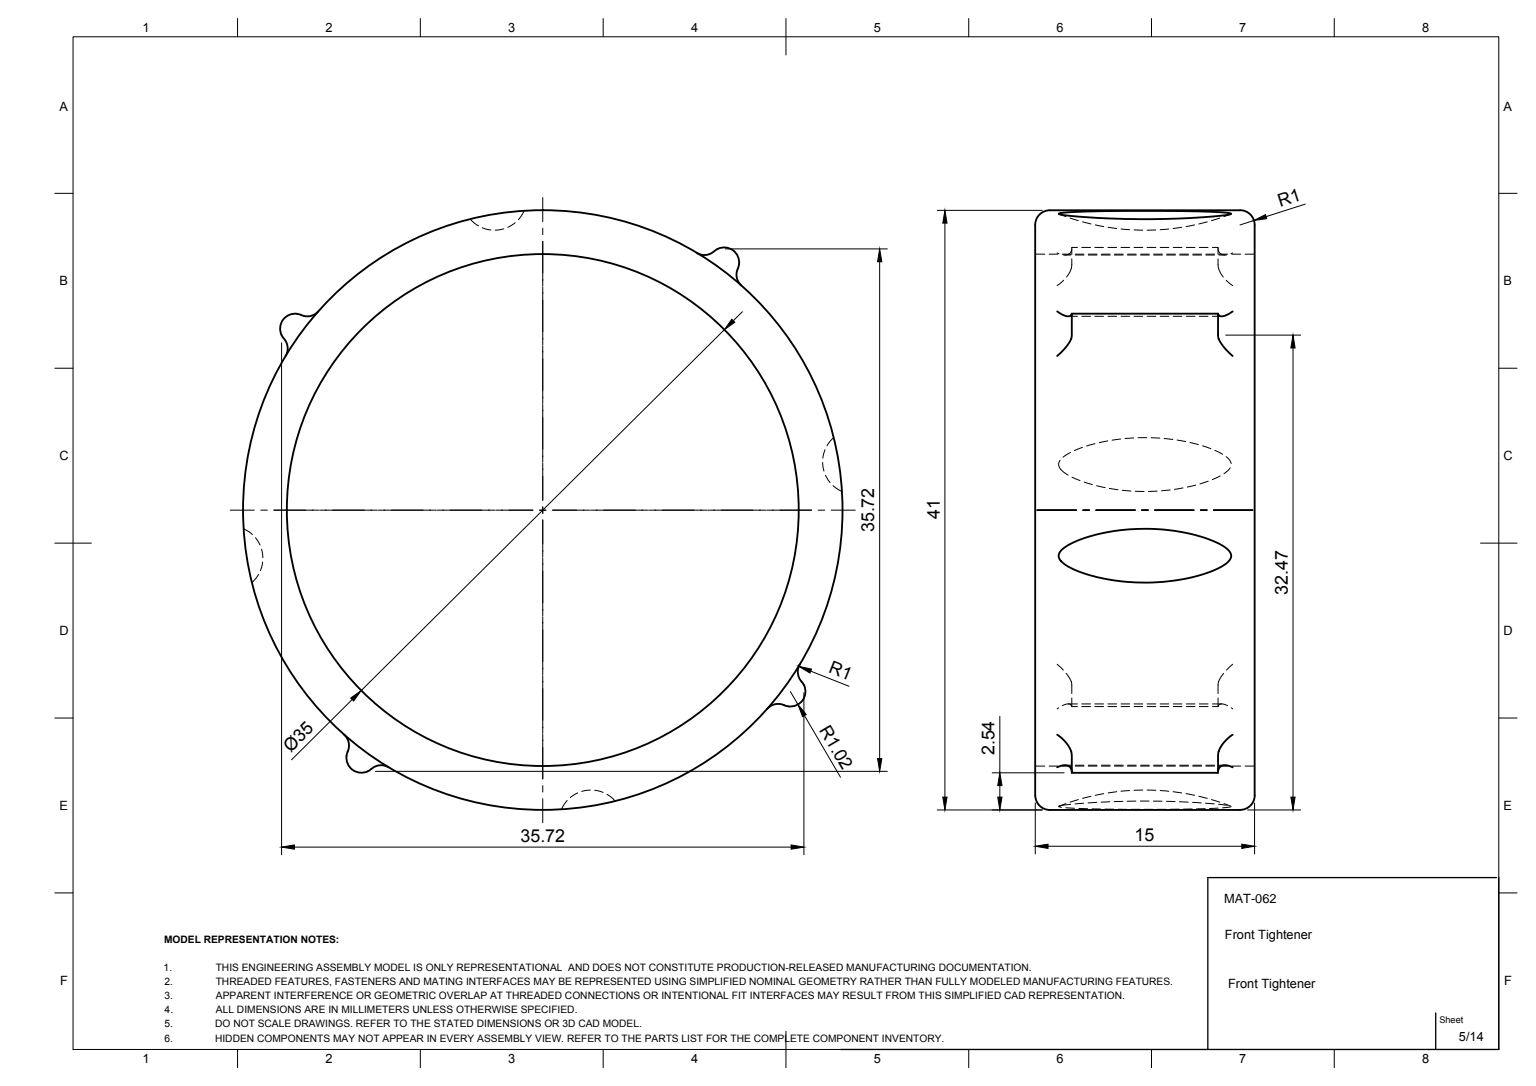
ISO-10303-21;
HEADER;
/* Generated by software containing ST-Developer
 * from STEP Tools, Inc. (www.steptools.com) 
 */

FILE_DESCRIPTION(
/* description */ (''),
/* implementation_level */ '2;1');

FILE_NAME(
/* name */ 'Front Tightener.step',
/* time_stamp */ '2026-10-24T10:18:25-07:00',
/* author */ (''),
/* organization */ (''),
/* preprocessor_version */ 'ST-DEVELOPER v20.2',
/* originating_system */ 'Autodesk Translation Framework v15.15.0.0',
/* authorisation */ '');

FILE_SCHEMA (('AUTOMOTIVE_DESIGN { 1 0 10303 214 3 1 1 }'));
ENDSEC;

DATA;
#10=MECHANICAL_DESIGN_GEOMETRIC_PRESENTATION_REPRESENTATION('',(#249),#14125);
#209=TOROIDAL_SURFACE('',#6436,21.5,1.);
#210=TOROIDAL_SURFACE('',#6437,21.5,1.);
#211=TOROIDAL_SURFACE('',#6461,21.5,1.);
#212=TOROIDAL_SURFACE('',#6462,21.5,1.);
#213=TOROIDAL_SURFACE('',#6465,21.5,1.);
#214=TOROIDAL_SURFACE('',#6466,21.5,1.);
#215=TOROIDAL_SURFACE('',#6469,21.5,1.);
#216=TOROIDAL_SURFACE('',#6470,21.5,1.);
#217=TOROIDAL_SURFACE('',#6472,19.5,1.);
#218=TOROIDAL_SURFACE('',#6474,19.5,1.);
#223=(
BOUNDED_SURFACE()
B_SPLINE_SURFACE(2,2,((#11091,#11092,#11093,#11094,#11095),(#11096,#11097,
#11098,#11099,#11100),(#11101,#11102,#11103,#11104,#11105)),
 .UNSPECIFIED.,.F.,.F.,.F.)
B_SPLINE_SURFACE_WITH_KNOTS((3,3),(3,2,3),(-0.372145961557786,0.372122372471418),
(-2.5862005619648,-1.57539112175776,-0.564581681550713),.UNSPECIFIED.)
GEOMETRIC_REPRESENTATION_ITEM()
RATIONAL_B_SPLINE_SURFACE(((1.,0.874978596158143,1.,0.874978596158143,1.),
(0.931553475244656,0.815089352015808,0.931553475244656,0.815089352015808,
0.931553475244656),(1.,0.874978596158143,1.,0.874978596158143,1.)))
REPRESENTATION_ITEM('')
SURFACE()
);
#224=(
BOUNDED_SURFACE()
B_SPLINE_SURFACE(2,2,((#11106,#11107,#11108,#11109,#11110),(#11111,#11112,
#11113,#11114,#11115),(#11116,#11117,#11118,#11119,#11120)),
 .UNSPECIFIED.,.F.,.F.,.F.)
B_SPLINE_SURFACE_WITH_KNOTS((3,3),(3,2,3),(-0.372145961557785,0.372122372471416),
(-1.01540423516984,-0.00459479496282911,1.00621464524418),.UNSPECIFIED.)
GEOMETRIC_REPRESENTATION_ITEM()
RATIONAL_B_SPLINE_SURFACE(((1.,0.874978596158151,1.,0.874978596158151,1.),
(0.931553475244656,0.815089352015816,0.931553475244656,0.815089352015816,
0.931553475244656),(1.,0.874978596158151,1.,0.874978596158151,1.)))
REPRESENTATION_ITEM('')
SURFACE()
);
#225=(
BOUNDED_SURFACE()
B_SPLINE_SURFACE(2,2,((#11121,#11122,#11123,#11124,#11125),(#11126,#11127,
#11128,#11129,#11130),(#11131,#11132,#11133,#11134,#11135)),
 .UNSPECIFIED.,.F.,.F.,.F.)
B_SPLINE_SURFACE_WITH_KNOTS((3,3),(3,2,3),(-0.372145961557786,0.372122372471418),
(0.555392091624955,1.56620153183202,2.57701097203908),.UNSPECIFIED.)
GEOMETRIC_REPRESENTATION_ITEM()
RATIONAL_B_SPLINE_SURFACE(((1.,0.874978596158138,1.,0.874978596158138,1.),
(0.931553475244654,0.815089352015803,0.931553475244654,0.815089352015803,
0.931553475244654),(1.,0.874978596158138,1.,0.874978596158138,1.)))
REPRESENTATION_ITEM('')
SURFACE()
);
#226=(
BOUNDED_SURFACE()
B_SPLINE_SURFACE(2,2,((#11136,#11137,#11138,#11139,#11140),(#11141,#11142,
#11143,#11144,#11145),(#11146,#11147,#11148,#11149,#11150)),
 .UNSPECIFIED.,.F.,.F.,.F.)
B_SPLINE_SURFACE_WITH_KNOTS((3,3),(3,2,3),(-0.371934671474245,0.371934671474244),
(-1.01080944020701,0.,1.01080944020701),.UNSPECIFIED.)
GEOMETRIC_REPRESENTATION_ITEM()
RATIONAL_B_SPLINE_SURFACE(((1.,0.87497859615815,1.,0.87497859615815,1.),
(0.93162599415309,0.815152804508512,0.93162599415309,0.815152804508512,
0.93162599415309),(1.,0.87497859615815,1.,0.87497859615815,1.)))
REPRESENTATION_ITEM('')
SURFACE()
);
#229=SHAPE_REPRESENTATION_RELATIONSHIP('SRR','None',#14202,#239);
#239=ADVANCED_BREP_SHAPE_REPRESENTATION('',(#268),#14116);
#249=STYLED_ITEM('',(#14263),#268);
#268=MANIFOLD_SOLID_BREP('Front Tightener',#6136);
#357=B_SPLINE_CURVE_WITH_KNOTS('',3,(#10853,#10854,#10855,#10856,#10857,
#10858,#10859,#10860),.UNSPECIFIED.,.F.,.F.,(4,2,2,4),(-1.01270550863141,
-0.972225883052009,-0.93592471729076,-0.9302261633243),.UNSPECIFIED.);
#358=B_SPLINE_CURVE_WITH_KNOTS('',3,(#10862,#10863,#10864,#10865,#10866,
#10867,#10868,#10869,#10870,#10871,#10872,#10873,#10874,#10875,#10876,#10877,
#10878,#10879,#10880,#10881,#10882,#10883),.UNSPECIFIED.,.F.,.F.,(4,2,2,
2,2,2,2,2,2,2,4),(0.770301299294677,0.776837516381544,0.810179859704117,
0.863854547164407,0.965601485426607,1.16658222290299,1.71041595764289,2.04547866914785,
2.21675572625692,2.31744906128486,2.32707423972487),.UNSPECIFIED.);
#359=B_SPLINE_CURVE_WITH_KNOTS('',3,(#10889,#10890,#10891,#10892,#10893,
#10894,#10895,#10896,#10897,#10898,#10899,#10900,#10901,#10902,#10903,#10904,
#10905,#10906,#10907,#10908,#10909,#10910,#10911,#10912,#10913),
 .UNSPECIFIED.,.F.,.F.,(4,2,2,2,2,3,2,2,2,2,2,4),(-0.9302261633243,-0.897559179923855,
-0.841033612998941,-0.72014052841894,-0.534875041413907,0.,0.287237711284631,
0.543909079429507,0.657892073847931,0.715678915934471,0.748705009105826,
0.770301299294677),.UNSPECIFIED.);
#360=B_SPLINE_CURVE_WITH_KNOTS('',3,(#10947,#10948,#10949,#10950,#10951,
#10952,#10953,#10954,#10955,#10956,#10957,#10958,#10959,#10960,#10961,#10962,
#10963,#10964,#10965,#10966,#10967,#10968,#10969,#10970,#10971,#10972,#10973,
#10974,#10975,#10976,#10977,#10978,#10979,#10980,#10981,#10982,#10983,#10984,
#10985,#10986,#10987,#10988,#10989,#10990),.UNSPECIFIED.,.T.,.F.,(4,2,2,
2,2,2,2,2,2,2,2,2,2,2,2,2,2,2,2,2,2,4),(-3.33977974833692,-3.05254203705232,
-2.79587066890727,-2.68188767448872,-2.62410083240212,-2.59107473923068,
-2.56294223195498,-2.52959988863245,-2.47592520117237,-2.37417826291126,
-2.17319752543706,-1.62936379070288,-1.29430107920164,-1.12302402209434,
-1.02233068706724,-0.972225883048282,-0.935924717287512,-0.897559179921191,
-0.841033612997187,-0.720140528418584,-0.534875041413949,0.),
 .UNSPECIFIED.);
#361=B_SPLINE_CURVE_WITH_KNOTS('',3,(#10992,#10993,#10994,#10995,#10996,
#10997,#10998,#10999,#11000,#11001,#11002,#11003,#11004,#11005,#11006,#11007,
#11008,#11009,#11010,#11011,#11012,#11013,#11014,#11015,#11016,#11017,#11018,
#11019,#11020,#11021,#11022,#11023,#11024,#11025,#11026,#11027,#11028,#11029,
#11030,#11031,#11032,#11033,#11034,#11035),.UNSPECIFIED.,.T.,.F.,(4,2,2,
2,2,2,2,2,2,2,2,2,2,2,2,2,2,2,2,2,2,4),(-3.3397797483622,-3.05254203707762,
-2.79587066893242,-2.68188767451365,-2.62410083242683,-2.5910747392553,
-2.5629422319795,-2.52959988865681,-2.47592520119621,-2.37417826293345,
-2.17319752545607,-1.62936379071395,-1.29430107920719,-1.1230240220981,
-1.02233068707054,-0.972225883051298,-0.93592471729009,-0.89755917992317,
-0.841033612998203,-0.720140528418294,-0.534875041413579,0.),
 .UNSPECIFIED.);
#362=B_SPLINE_CURVE_WITH_KNOTS('',3,(#11037,#11038,#11039,#11040,#11041,
#11042,#11043,#11044,#11045,#11046,#11047,#11048,#11049,#11050,#11051,#11052,
#11053,#11054,#11055,#11056,#11057,#11058,#11059,#11060,#11061,#11062,#11063,
#11064,#11065,#11066,#11067,#11068,#11069,#11070,#11071,#11072,#11073,#11074,
#11075,#11076,#11077,#11078,#11079,#11080),.UNSPECIFIED.,.T.,.F.,(4,2,2,
2,2,2,2,2,2,2,2,2,2,2,2,2,2,2,2,2,2,4),(-3.3397797483903,-3.05254203710569,
-2.79587066896086,-2.68188767454252,-2.62410083245608,-2.59107473928483,
-2.56294223200934,-2.52959988868709,-2.47592520122646,-2.37417826296174,
-2.17319752548078,-1.62936379072977,-1.29430107921846,-1.12302402210607,
-1.02233068707609,-0.972225883055856,-0.935924717293985,-0.897559179926439,
-0.841033613000712,-0.720140528419696,-0.534875041414283,0.),
 .UNSPECIFIED.);
#363=B_SPLINE_CURVE_WITH_KNOTS('',3,(#11156,#11157,#11158,#11159,#11160,
#11161),.UNSPECIFIED.,.F.,.F.,(4,2,4),(0.661047189651573,0.682893822496354,
0.69260663288377),.UNSPECIFIED.);
#364=B_SPLINE_CURVE_WITH_KNOTS('',3,(#11165,#11166,#11167,#11168,#11169,
#11170),.UNSPECIFIED.,.F.,.F.,(4,2,4),(0.954385955540414,0.955688960187291,
0.983990255335198),.UNSPECIFIED.);
#365=B_SPLINE_CURVE_WITH_KNOTS('',3,(#11174,#11175,#11176,#11177,#11178,
#11179),.UNSPECIFIED.,.F.,.F.,(4,2,4),(0.11431583352954,0.135832218753253,
0.145774815807224),.UNSPECIFIED.);
#366=B_SPLINE_CURVE_WITH_KNOTS('',3,(#11182,#11183,#11184,#11185,#11186,
#11187),.UNSPECIFIED.,.F.,.F.,(4,2,4),(0.406957049146252,0.408029153839697,
0.43652027355868),.UNSPECIFIED.);
#367=B_SPLINE_CURVE_WITH_KNOTS('',3,(#11193,#11194,#11195,#11196,#11197,
#11198,#11199,#11200,#11201,#11202),.UNSPECIFIED.,.F.,.F.,(4,2,2,2,4),(-0.178698063821344,
-0.13526955955559,-0.076624980274606,0.,0.000624348927189005),
 .UNSPECIFIED.);
#368=B_SPLINE_CURVE_WITH_KNOTS('',3,(#11203,#11204,#11205,#11206,#11207,
#11208,#11209,#11210,#11211,#11212),.UNSPECIFIED.,.F.,.F.,(4,2,2,2,4),(0.221433756193381,
0.257003031040665,0.305034737267452,0.367792942517405,0.3683043034075),
 .UNSPECIFIED.);
#369=B_SPLINE_CURVE_WITH_KNOTS('',3,(#11214,#11215,#11216,#11217,#11218,
#11219,#11220,#11221,#11222,#11223),.UNSPECIFIED.,.F.,.F.,(4,2,2,2,4),(-0.178698063657826,
-0.135269559443281,-0.0766249802302674,0.,0.000624348926984052),
 .UNSPECIFIED.);
#370=B_SPLINE_CURVE_WITH_KNOTS('',3,(#11225,#11226,#11227,#11228,#11229,
#11230,#11231,#11232,#11233,#11234),.UNSPECIFIED.,.F.,.F.,(4,2,2,2,4),(0.22143375619356,
0.257003031040236,0.305034737266783,0.367792942534155,0.36830430342492),
 .UNSPECIFIED.);
#371=B_SPLINE_CURVE_WITH_KNOTS('',3,(#11241,#11242,#11243,#11244,#11245,
#11246),.UNSPECIFIED.,.F.,.F.,(4,2,4),(0.661047189631137,0.682893822475484,
0.692606632862655),.UNSPECIFIED.);
#372=B_SPLINE_CURVE_WITH_KNOTS('',3,(#11250,#11251,#11252,#11253,#11254,
#11255),.UNSPECIFIED.,.F.,.F.,(4,2,4),(0.954385955875588,0.955688960523108,
0.983990255684603),.UNSPECIFIED.);
#373=B_SPLINE_CURVE_WITH_KNOTS('',3,(#11259,#11260,#11261,#11262,#11263,
#11264),.UNSPECIFIED.,.F.,.F.,(4,2,4),(0.11431583355748,0.135832218786672,
0.145774815843186),.UNSPECIFIED.);
#374=B_SPLINE_CURVE_WITH_KNOTS('',3,(#11267,#11268,#11269,#11270,#11271,
#11272),.UNSPECIFIED.,.F.,.F.,(4,2,4),(0.406957049130622,0.408029153824045,
0.436520273542523),.UNSPECIFIED.);
#375=B_SPLINE_CURVE_WITH_KNOTS('',3,(#11282,#11283,#11284,#11285,#11286,
#11287),.UNSPECIFIED.,.F.,.F.,(4,2,4),(0.661047189621191,0.682893822464398,
0.692606632851314),.UNSPECIFIED.);
#376=B_SPLINE_CURVE_WITH_KNOTS('',3,(#11291,#11292,#11293,#11294,#11295,
#11296),.UNSPECIFIED.,.F.,.F.,(4,2,4),(0.954385955650832,0.95568896029806,
0.983990255452134),.UNSPECIFIED.);
#377=B_SPLINE_CURVE_WITH_KNOTS('',3,(#11300,#11301,#11302,#11303,#11304,
#11305),.UNSPECIFIED.,.F.,.F.,(4,2,4),(0.114315833531678,0.135832218756235,
0.145774815810657),.UNSPECIFIED.);
#378=B_SPLINE_CURVE_WITH_KNOTS('',3,(#11308,#11309,#11310,#11311,#11312,
#11313),.UNSPECIFIED.,.F.,.F.,(4,2,4),(0.406957049123385,0.408029153816832,
0.43652027353595),.UNSPECIFIED.);
#379=B_SPLINE_CURVE_WITH_KNOTS('',3,(#11323,#11324,#11325,#11326,#11327,
#11328),.UNSPECIFIED.,.F.,.F.,(4,2,4),(0.661047189700789,0.682893822549002,
0.692606632937976),.UNSPECIFIED.);
#380=B_SPLINE_CURVE_WITH_KNOTS('',3,(#11332,#11333,#11334,#11335,#11336,
#11337),.UNSPECIFIED.,.F.,.F.,(4,2,4),(0.954385955972242,0.955688960619816,
0.983990255786846),.UNSPECIFIED.);
#381=B_SPLINE_CURVE_WITH_KNOTS('',3,(#11341,#11342,#11343,#11344,#11345,
#11346),.UNSPECIFIED.,.F.,.F.,(4,2,4),(0.114315833560946,0.135832218791008,
0.145774815847966),.UNSPECIFIED.);
#382=B_SPLINE_CURVE_WITH_KNOTS('',3,(#11349,#11350,#11351,#11352,#11353,
#11354),.UNSPECIFIED.,.F.,.F.,(4,2,4),(0.406957049170082,0.408029153863569,
0.436520273584039),.UNSPECIFIED.);
#383=B_SPLINE_CURVE_WITH_KNOTS('',3,(#11360,#11361,#11362,#11363,#11364,
#11365,#11366,#11367,#11368,#11369),.UNSPECIFIED.,.F.,.F.,(4,2,2,2,4),(-0.17869806353704,
-0.135269559359834,-0.0766249801970823,0.,0.000624348926732177),
 .UNSPECIFIED.);
#384=B_SPLINE_CURVE_WITH_KNOTS('',3,(#11370,#11371,#11372,#11373,#11374,
#11375,#11376,#11377,#11378,#11379),.UNSPECIFIED.,.F.,.F.,(4,2,2,2,4),(0.221433756192697,
0.257003031038445,0.305034737264325,0.3677929425703,0.368304303461073),
 .UNSPECIFIED.);
#385=B_SPLINE_CURVE_WITH_KNOTS('',3,(#11381,#11382,#11383,#11384,#11385,
#11386,#11387,#11388,#11389,#11390),.UNSPECIFIED.,.F.,.F.,(4,2,2,2,4),(-0.178698063770044,
-0.135269559520182,-0.0766249802604931,0.,0.000624348926843672),
 .UNSPECIFIED.);
#386=B_SPLINE_CURVE_WITH_KNOTS('',3,(#11392,#11393,#11394,#11395,#11396,
#11397,#11398,#11399,#11400,#11401),.UNSPECIFIED.,.F.,.F.,(4,2,2,2,4),(0.221433756193478,
0.257003031040149,0.305034737266569,0.367792942538401,0.368304303428461),
 .UNSPECIFIED.);
#387=B_SPLINE_CURVE_WITH_KNOTS('',3,(#11404,#11405,#11406,#11407,#11408,
#11409,#11410,#11411,#11412,#11413),.UNSPECIFIED.,.F.,.F.,(4,2,2,2,4),(-0.178698063553284,
-0.135269559371072,-0.0766249802015666,0.,0.000624348926677296),
 .UNSPECIFIED.);
#388=B_SPLINE_CURVE_WITH_KNOTS('',3,(#11414,#11415,#11416,#11417,#11418,
#11419,#11420,#11421,#11422,#11423),.UNSPECIFIED.,.F.,.F.,(4,2,2,2,4),(0.221433756192838,
0.25700303103897,0.305034737265084,0.367792942555533,0.368304303445851),
 .UNSPECIFIED.);
#389=B_SPLINE_CURVE_WITH_KNOTS('',3,(#11425,#11426,#11427,#11428,#11429,
#11430,#11431,#11432,#11433,#11434),.UNSPECIFIED.,.F.,.F.,(4,2,2,2,4),(-0.178698063553173,
-0.135269559370956,-0.0766249802014978,0.,0.000624348926817562),
 .UNSPECIFIED.);
#390=B_SPLINE_CURVE_WITH_KNOTS('',3,(#11436,#11437,#11438,#11439,#11440,
#11441,#11442,#11443,#11444,#11445),.UNSPECIFIED.,.F.,.F.,(4,2,2,2,4),(0.221433756193333,
0.25700303103906,0.305034737264906,0.367792942572609,0.368304303463133),
 .UNSPECIFIED.);
#391=B_SPLINE_CURVE_WITH_KNOTS('',3,(#11448,#11449,#11450,#11451,#11452,
#11453,#11454,#11455,#11456,#11457),.UNSPECIFIED.,.F.,.F.,(4,2,2,2,4),(-0.178698063530463,
-0.135269559355353,-0.0766249801953056,0.,0.000624348926771406),
 .UNSPECIFIED.);
#392=B_SPLINE_CURVE_WITH_KNOTS('',3,(#11458,#11459,#11460,#11461,#11462,
#11463,#11464,#11465,#11466,#11467),.UNSPECIFIED.,.F.,.F.,(4,2,2,2,4),(0.221433756193692,
0.2570030310401,0.30503473726647,0.367792942548679,0.368304303439319),
 .UNSPECIFIED.);
#393=B_SPLINE_CURVE_WITH_KNOTS('',3,(#11469,#11470,#11471,#11472,#11473,
#11474,#11475,#11476,#11477,#11478),.UNSPECIFIED.,.F.,.F.,(4,2,2,2,4),(-0.178698063395802,
-0.135269559262804,-0.0766249801587596,0.,0.00062434892634055),
 .UNSPECIFIED.);
#394=B_SPLINE_CURVE_WITH_KNOTS('',3,(#11480,#11481,#11482,#11483,#11484,
#11485,#11486,#11487,#11488,#11489),.UNSPECIFIED.,.F.,.F.,(4,2,2,2,4),(0.221433756192834,
0.257003031038388,0.305034737264263,0.367792942576978,0.368304303467952),
 .UNSPECIFIED.);
#513=CYLINDRICAL_SURFACE('',#6409,20.5);
#514=CYLINDRICAL_SURFACE('',#6428,1.02425693042952);
#515=CYLINDRICAL_SURFACE('',#6435,1.);
#516=CYLINDRICAL_SURFACE('',#6438,1.);
#517=CYLINDRICAL_SURFACE('',#6439,1.02425693042952);
#518=CYLINDRICAL_SURFACE('',#6446,1.02425693042952);
#519=CYLINDRICAL_SURFACE('',#6453,1.02425693042952);
#520=CYLINDRICAL_SURFACE('',#6460,1.);
#521=CYLINDRICAL_SURFACE('',#6463,1.);
#522=CYLINDRICAL_SURFACE('',#6464,1.);
#523=CYLINDRICAL_SURFACE('',#6467,1.);
#524=CYLINDRICAL_SURFACE('',#6468,1.);
#525=CYLINDRICAL_SURFACE('',#6471,1.);
#526=CYLINDRICAL_SURFACE('',#6476,17.5);
#654=FACE_BOUND('',#1203,.T.);
#655=FACE_BOUND('',#1204,.T.);
#656=FACE_BOUND('',#1205,.T.);
#657=FACE_BOUND('',#1206,.T.);
#658=FACE_BOUND('',#1207,.T.);
#659=FACE_BOUND('',#1208,.T.);
#660=FACE_BOUND('',#1209,.T.);
#661=FACE_BOUND('',#1211,.T.);
#662=FACE_BOUND('',#1213,.T.);
#822=FACE_OUTER_BOUND('',#1202,.T.);
#823=FACE_OUTER_BOUND('',#1210,.T.);
#824=FACE_OUTER_BOUND('',#1212,.T.);
#825=FACE_OUTER_BOUND('',#1214,.T.);
#826=FACE_OUTER_BOUND('',#1215,.T.);
#827=FACE_OUTER_BOUND('',#1216,.T.);
#828=FACE_OUTER_BOUND('',#1217,.T.);
#829=FACE_OUTER_BOUND('',#1218,.T.);
#830=FACE_OUTER_BOUND('',#1219,.T.);
#831=FACE_OUTER_BOUND('',#1220,.T.);
#832=FACE_OUTER_BOUND('',#1221,.T.);
#833=FACE_OUTER_BOUND('',#1222,.T.);
#834=FACE_OUTER_BOUND('',#1223,.T.);
#835=FACE_OUTER_BOUND('',#1224,.T.);
#836=FACE_OUTER_BOUND('',#1225,.T.);
#837=FACE_OUTER_BOUND('',#1226,.T.);
#838=FACE_OUTER_BOUND('',#1227,.T.);
#839=FACE_OUTER_BOUND('',#1228,.T.);
#840=FACE_OUTER_BOUND('',#1229,.T.);
#841=FACE_OUTER_BOUND('',#1230,.T.);
#842=FACE_OUTER_BOUND('',#1231,.T.);
#843=FACE_OUTER_BOUND('',#1232,.T.);
#844=FACE_OUTER_BOUND('',#1233,.T.);
#845=FACE_OUTER_BOUND('',#1234,.T.);
#846=FACE_OUTER_BOUND('',#1235,.T.);
#847=FACE_OUTER_BOUND('',#1236,.T.);
#848=FACE_OUTER_BOUND('',#1237,.T.);
#849=FACE_OUTER_BOUND('',#1238,.T.);
#850=FACE_OUTER_BOUND('',#1239,.T.);
#851=FACE_OUTER_BOUND('',#1240,.T.);
#852=FACE_OUTER_BOUND('',#1241,.T.);
#853=FACE_OUTER_BOUND('',#1242,.T.);
#854=FACE_OUTER_BOUND('',#1243,.T.);
#855=FACE_OUTER_BOUND('',#1244,.T.);
#856=FACE_OUTER_BOUND('',#1245,.T.);
#857=FACE_OUTER_BOUND('',#1246,.T.);
#858=FACE_OUTER_BOUND('',#1247,.T.);
#859=FACE_OUTER_BOUND('',#1248,.T.);
#1202=EDGE_LOOP('',(#4403,#4404,#4405,#4406,#4407,#4408,#4409,#4410,#4411,
#4412,#4413));
#1203=EDGE_LOOP('',(#4414,#4415,#4416,#4417));
#1204=EDGE_LOOP('',(#4418,#4419,#4420,#4421));
#1205=EDGE_LOOP('',(#4422,#4423,#4424,#4425));
#1206=EDGE_LOOP('',(#4426,#4427,#4428,#4429));
#1207=EDGE_LOOP('',(#4430));
#1208=EDGE_LOOP('',(#4431));
#1209=EDGE_LOOP('',(#4432));
#1210=EDGE_LOOP('',(#4433));
#1211=EDGE_LOOP('',(#4434));
#1212=EDGE_LOOP('',(#4435));
#1213=EDGE_LOOP('',(#4436));
#1214=EDGE_LOOP('',(#4437));
#1215=EDGE_LOOP('',(#4438));
#1216=EDGE_LOOP('',(#4439));
#1217=EDGE_LOOP('',(#4440,#4441,#4442));
#1218=EDGE_LOOP('',(#4443,#4444,#4445,#4446,#4447,#4448,#4449,#4450));
#1219=EDGE_LOOP('',(#4451,#4452));
#1220=EDGE_LOOP('',(#4453,#4454));
#1221=EDGE_LOOP('',(#4455,#4456,#4457,#4458));
#1222=EDGE_LOOP('',(#4459,#4460,#4461,#4462,#4463,#4464));
#1223=EDGE_LOOP('',(#4465,#4466,#4467,#4468,#4469,#4470));
#1224=EDGE_LOOP('',(#4471,#4472,#4473,#4474));
#1225=EDGE_LOOP('',(#4475,#4476,#4477,#4478,#4479,#4480,#4481,#4482));
#1226=EDGE_LOOP('',(#4483,#4484));
#1227=EDGE_LOOP('',(#4485,#4486));
#1228=EDGE_LOOP('',(#4487,#4488,#4489,#4490,#4491,#4492,#4493,#4494));
#1229=EDGE_LOOP('',(#4495,#4496));
#1230=EDGE_LOOP('',(#4497,#4498));
#1231=EDGE_LOOP('',(#4499,#4500,#4501,#4502,#4503,#4504,#4505,#4506));
#1232=EDGE_LOOP('',(#4507,#4508));
#1233=EDGE_LOOP('',(#4509,#4510));
#1234=EDGE_LOOP('',(#4511,#4512,#4513,#4514));
#1235=EDGE_LOOP('',(#4515,#4516,#4517,#4518,#4519,#4520));
#1236=EDGE_LOOP('',(#4521,#4522,#4523,#4524,#4525,#4526));
#1237=EDGE_LOOP('',(#4527,#4528,#4529,#4530));
#1238=EDGE_LOOP('',(#4531,#4532,#4533,#4534));
#1239=EDGE_LOOP('',(#4535,#4536,#4537,#4538,#4539,#4540));
#1240=EDGE_LOOP('',(#4541,#4542,#4543,#4544,#4545,#4546));
#1241=EDGE_LOOP('',(#4547,#4548,#4549,#4550));
#1242=EDGE_LOOP('',(#4551,#4552,#4553,#4554));
#1243=EDGE_LOOP('',(#4555,#4556,#4557,#4558,#4559,#4560));
#1244=EDGE_LOOP('',(#4561,#4562,#4563,#4564,#4565,#4566));
#1245=EDGE_LOOP('',(#4567,#4568,#4569,#4570));
#1246=EDGE_LOOP('',(#4571,#4572,#4573,#4574,#4575));
#1247=EDGE_LOOP('',(#4576,#4577,#4578,#4579,#4580));
#1248=EDGE_LOOP('',(#4581,#4582,#4583,#4584));
#1614=CIRCLE('',#6410,20.5);
#1615=CIRCLE('',#6411,20.5);
#1616=CIRCLE('',#6412,20.5);
#1617=CIRCLE('',#6413,20.5);
#1618=CIRCLE('',#6414,20.5);
#1619=CIRCLE('',#6415,20.5);
#1620=CIRCLE('',#6416,20.5);
#1621=CIRCLE('',#6417,20.5);
#1622=CIRCLE('',#6418,20.5);
#1623=CIRCLE('',#6419,20.5);
#1624=CIRCLE('',#6420,20.5);
#1625=CIRCLE('',#6421,20.5);
#1626=CIRCLE('',#6423,19.5);
#1627=CIRCLE('',#6424,17.5);
#1628=CIRCLE('',#6426,19.5);
#1629=CIRCLE('',#6427,17.5);
#1630=CIRCLE('',#6429,1.02425693042952);
#1631=CIRCLE('',#6430,1.02425693042952);
#1632=CIRCLE('',#6432,21.5);
#1633=CIRCLE('',#6434,21.5);
#1634=CIRCLE('',#6440,1.02425693042952);
#1635=CIRCLE('',#6441,1.02425693042952);
#1636=CIRCLE('',#6443,21.5);
#1637=CIRCLE('',#6445,21.5);
#1638=CIRCLE('',#6447,1.02425693042952);
#1639=CIRCLE('',#6448,1.02425693042952);
#1640=CIRCLE('',#6450,21.5);
#1641=CIRCLE('',#6452,21.5);
#1642=CIRCLE('',#6454,1.02425693042952);
#1643=CIRCLE('',#6455,1.02425693042952);
#1644=CIRCLE('',#6457,21.5);
#1645=CIRCLE('',#6459,21.5);
#1646=CIRCLE('',#6473,1.);
#1647=CIRCLE('',#6475,1.);
#1888=LINE('',#10851,#2276);
#1889=LINE('',#10885,#2277);
#1890=LINE('',#10916,#2278);
#1891=LINE('',#10920,#2279);
#1892=LINE('',#10924,#2280);
#1893=LINE('',#10928,#2281);
#1894=LINE('',#10932,#2282);
#1895=LINE('',#10936,#2283);
#1896=LINE('',#10940,#2284);
#1897=LINE('',#10944,#2285);
#1898=LINE('',#11163,#2286);
#1899=LINE('',#11181,#2287);
#1900=LINE('',#11248,#2288);
#1901=LINE('',#11266,#2289);
#1902=LINE('',#11289,#2290);
#1903=LINE('',#11307,#2291);
#1904=LINE('',#11330,#2292);
#1905=LINE('',#11348,#2293);
#1906=LINE('',#11496,#2294);
#2276=VECTOR('',#7300,20.5);
#2277=VECTOR('',#7301,20.5);
#2278=VECTOR('',#7306,12.);
#2279=VECTOR('',#7309,12.);
#2280=VECTOR('',#7312,12.);
#2281=VECTOR('',#7315,12.);
#2282=VECTOR('',#7318,12.);
#2283=VECTOR('',#7321,12.);
#2284=VECTOR('',#7324,12.);
#2285=VECTOR('',#7327,12.);
#2286=VECTOR('',#7346,10.0757988598381);
#2287=VECTOR('',#7349,10.0757988598381);
#2288=VECTOR('',#7370,10.0757988598381);
#2289=VECTOR('',#7373,10.0757988598381);
#2290=VECTOR('',#7386,10.0757988598381);
#2291=VECTOR('',#7389,10.0757988598381);
#2292=VECTOR('',#7402,10.0757988598381);
#2293=VECTOR('',#7405,10.0757988598381);
#2294=VECTOR('',#7448,17.5);
#2721=VERTEX_POINT('',#10846);
#2722=VERTEX_POINT('',#10847);
#2723=VERTEX_POINT('',#10850);
#2724=VERTEX_POINT('',#10852);
#2725=VERTEX_POINT('',#10861);
#2726=VERTEX_POINT('',#10884);
#2727=VERTEX_POINT('',#10886);
#2728=VERTEX_POINT('',#10914);
#2729=VERTEX_POINT('',#10915);
#2730=VERTEX_POINT('',#10917);
#2731=VERTEX_POINT('',#10919);
#2732=VERTEX_POINT('',#10922);
#2733=VERTEX_POINT('',#10923);
#2734=VERTEX_POINT('',#10925);
#2735=VERTEX_POINT('',#10927);
#2736=VERTEX_POINT('',#10930);
#2737=VERTEX_POINT('',#10931);
#2738=VERTEX_POINT('',#10933);
#2739=VERTEX_POINT('',#10935);
#2740=VERTEX_POINT('',#10938);
#2741=VERTEX_POINT('',#10939);
#2742=VERTEX_POINT('',#10941);
#2743=VERTEX_POINT('',#10943);
#2744=VERTEX_POINT('',#10946);
#2745=VERTEX_POINT('',#10991);
#2746=VERTEX_POINT('',#11036);
#2747=VERTEX_POINT('',#11082);
#2748=VERTEX_POINT('',#11084);
#2749=VERTEX_POINT('',#11087);
#2750=VERTEX_POINT('',#11089);
#2751=VERTEX_POINT('',#11152);
#2752=VERTEX_POINT('',#11153);
#2753=VERTEX_POINT('',#11155);
#2754=VERTEX_POINT('',#11162);
#2755=VERTEX_POINT('',#11164);
#2756=VERTEX_POINT('',#11171);
#2757=VERTEX_POINT('',#11173);
#2758=VERTEX_POINT('',#11180);
#2759=VERTEX_POINT('',#11237);
#2760=VERTEX_POINT('',#11238);
#2761=VERTEX_POINT('',#11240);
#2762=VERTEX_POINT('',#11247);
#2763=VERTEX_POINT('',#11249);
#2764=VERTEX_POINT('',#11256);
#2765=VERTEX_POINT('',#11258);
#2766=VERTEX_POINT('',#11265);
#2767=VERTEX_POINT('',#11278);
#2768=VERTEX_POINT('',#11279);
#2769=VERTEX_POINT('',#11281);
#2770=VERTEX_POINT('',#11288);
#2771=VERTEX_POINT('',#11290);
#2772=VERTEX_POINT('',#11297);
#2773=VERTEX_POINT('',#11299);
#2774=VERTEX_POINT('',#11306);
#2775=VERTEX_POINT('',#11319);
#2776=VERTEX_POINT('',#11320);
#2777=VERTEX_POINT('',#11322);
#2778=VERTEX_POINT('',#11329);
#2779=VERTEX_POINT('',#11331);
#2780=VERTEX_POINT('',#11338);
#2781=VERTEX_POINT('',#11340);
#2782=VERTEX_POINT('',#11347);
#3349=EDGE_CURVE('',#2721,#2722,#1614,.T.);
#3350=EDGE_CURVE('',#2722,#2721,#1615,.T.);
#3351=EDGE_CURVE('',#2721,#2723,#1888,.T.);
#3352=EDGE_CURVE('',#2724,#2723,#357,.T.);
#3353=EDGE_CURVE('',#2725,#2724,#358,.T.);
#3354=EDGE_CURVE('',#2725,#2726,#1889,.T.);
#3355=EDGE_CURVE('',#2726,#2727,#1616,.F.);
#3356=EDGE_CURVE('',#2727,#2726,#1617,.F.);
#3357=EDGE_CURVE('',#2723,#2725,#359,.T.);
#3358=EDGE_CURVE('',#2728,#2729,#1890,.F.);
#3359=EDGE_CURVE('',#2729,#2730,#1618,.T.);
#3360=EDGE_CURVE('',#2730,#2731,#1891,.T.);
#3361=EDGE_CURVE('',#2731,#2728,#1619,.F.);
#3362=EDGE_CURVE('',#2732,#2733,#1892,.F.);
#3363=EDGE_CURVE('',#2733,#2734,#1620,.T.);
#3364=EDGE_CURVE('',#2734,#2735,#1893,.T.);
#3365=EDGE_CURVE('',#2735,#2732,#1621,.F.);
#3366=EDGE_CURVE('',#2736,#2737,#1894,.F.);
#3367=EDGE_CURVE('',#2737,#2738,#1622,.T.);
#3368=EDGE_CURVE('',#2738,#2739,#1895,.T.);
#3369=EDGE_CURVE('',#2739,#2736,#1623,.F.);
#3370=EDGE_CURVE('',#2740,#2741,#1896,.F.);
#3371=EDGE_CURVE('',#2741,#2742,#1624,.T.);
#3372=EDGE_CURVE('',#2742,#2743,#1897,.T.);
#3373=EDGE_CURVE('',#2743,#2740,#1625,.F.);
#3374=EDGE_CURVE('',#2744,#2744,#360,.T.);
#3375=EDGE_CURVE('',#2745,#2745,#361,.T.);
#3376=EDGE_CURVE('',#2746,#2746,#362,.T.);
#3377=EDGE_CURVE('',#2747,#2747,#1626,.T.);
#3378=EDGE_CURVE('',#2748,#2748,#1627,.T.);
#3379=EDGE_CURVE('',#2749,#2749,#1628,.F.);
#3380=EDGE_CURVE('',#2750,#2750,#1629,.T.);
#3381=EDGE_CURVE('',#2751,#2752,#1630,.T.);
#3382=EDGE_CURVE('',#2751,#2753,#363,.T.);
#3383=EDGE_CURVE('',#2753,#2754,#1898,.T.);
#3384=EDGE_CURVE('',#2754,#2755,#364,.T.);
#3385=EDGE_CURVE('',#2755,#2756,#1631,.T.);
#3386=EDGE_CURVE('',#2756,#2757,#365,.T.);
#3387=EDGE_CURVE('',#2757,#2758,#1899,.F.);
#3388=EDGE_CURVE('',#2758,#2752,#366,.T.);
#3389=EDGE_CURVE('',#2752,#2751,#1632,.F.);
#3390=EDGE_CURVE('',#2755,#2756,#1633,.T.);
#3391=EDGE_CURVE('',#2743,#2757,#367,.F.);
#3392=EDGE_CURVE('',#2758,#2742,#368,.T.);
#3393=EDGE_CURVE('',#2753,#2741,#369,.T.);
#3394=EDGE_CURVE('',#2740,#2754,#370,.F.);
#3395=EDGE_CURVE('',#2759,#2760,#1634,.T.);
#3396=EDGE_CURVE('',#2759,#2761,#371,.T.);
#3397=EDGE_CURVE('',#2761,#2762,#1900,.T.);
#3398=EDGE_CURVE('',#2762,#2763,#372,.T.);
#3399=EDGE_CURVE('',#2763,#2764,#1635,.T.);
#3400=EDGE_CURVE('',#2764,#2765,#373,.T.);
#3401=EDGE_CURVE('',#2765,#2766,#1901,.F.);
#3402=EDGE_CURVE('',#2766,#2760,#374,.T.);
#3403=EDGE_CURVE('',#2760,#2759,#1636,.F.);
#3404=EDGE_CURVE('',#2763,#2764,#1637,.T.);
#3405=EDGE_CURVE('',#2767,#2768,#1638,.T.);
#3406=EDGE_CURVE('',#2767,#2769,#375,.T.);
#3407=EDGE_CURVE('',#2769,#2770,#1902,.T.);
#3408=EDGE_CURVE('',#2770,#2771,#376,.T.);
#3409=EDGE_CURVE('',#2771,#2772,#1639,.T.);
#3410=EDGE_CURVE('',#2772,#2773,#377,.T.);
#3411=EDGE_CURVE('',#2773,#2774,#1903,.F.);
#3412=EDGE_CURVE('',#2774,#2768,#378,.T.);
#3413=EDGE_CURVE('',#2768,#2767,#1640,.F.);
#3414=EDGE_CURVE('',#2771,#2772,#1641,.T.);
#3415=EDGE_CURVE('',#2775,#2776,#1642,.T.);
#3416=EDGE_CURVE('',#2775,#2777,#379,.T.);
#3417=EDGE_CURVE('',#2777,#2778,#1904,.T.);
#3418=EDGE_CURVE('',#2778,#2779,#380,.T.);
#3419=EDGE_CURVE('',#2779,#2780,#1643,.T.);
#3420=EDGE_CURVE('',#2780,#2781,#381,.T.);
#3421=EDGE_CURVE('',#2781,#2782,#1905,.F.);
#3422=EDGE_CURVE('',#2782,#2776,#382,.T.);
#3423=EDGE_CURVE('',#2776,#2775,#1644,.F.);
#3424=EDGE_CURVE('',#2779,#2780,#1645,.T.);
#3425=EDGE_CURVE('',#2739,#2781,#383,.F.);
#3426=EDGE_CURVE('',#2782,#2738,#384,.T.);
#3427=EDGE_CURVE('',#2777,#2737,#385,.T.);
#3428=EDGE_CURVE('',#2736,#2778,#386,.F.);
#3429=EDGE_CURVE('',#2735,#2773,#387,.F.);
#3430=EDGE_CURVE('',#2774,#2734,#388,.T.);
#3431=EDGE_CURVE('',#2769,#2733,#389,.T.);
#3432=EDGE_CURVE('',#2732,#2770,#390,.F.);
#3433=EDGE_CURVE('',#2731,#2765,#391,.F.);
#3434=EDGE_CURVE('',#2766,#2730,#392,.T.);
#3435=EDGE_CURVE('',#2761,#2729,#393,.T.);
#3436=EDGE_CURVE('',#2728,#2762,#394,.F.);
#3437=EDGE_CURVE('',#2722,#2749,#1646,.T.);
#3438=EDGE_CURVE('',#2747,#2727,#1647,.T.);
#3439=EDGE_CURVE('',#2750,#2748,#1906,.T.);
#4403=ORIENTED_EDGE('',*,*,#3349,.T.);
#4404=ORIENTED_EDGE('',*,*,#3350,.T.);
#4405=ORIENTED_EDGE('',*,*,#3351,.T.);
#4406=ORIENTED_EDGE('',*,*,#3352,.F.);
#4407=ORIENTED_EDGE('',*,*,#3353,.F.);
#4408=ORIENTED_EDGE('',*,*,#3354,.T.);
#4409=ORIENTED_EDGE('',*,*,#3355,.T.);
#4410=ORIENTED_EDGE('',*,*,#3356,.T.);
#4411=ORIENTED_EDGE('',*,*,#3354,.F.);
#4412=ORIENTED_EDGE('',*,*,#3357,.F.);
#4413=ORIENTED_EDGE('',*,*,#3351,.F.);
#4414=ORIENTED_EDGE('',*,*,#3358,.T.);
#4415=ORIENTED_EDGE('',*,*,#3359,.T.);
#4416=ORIENTED_EDGE('',*,*,#3360,.T.);
#4417=ORIENTED_EDGE('',*,*,#3361,.T.);
#4418=ORIENTED_EDGE('',*,*,#3362,.T.);
#4419=ORIENTED_EDGE('',*,*,#3363,.T.);
#4420=ORIENTED_EDGE('',*,*,#3364,.T.);
#4421=ORIENTED_EDGE('',*,*,#3365,.T.);
#4422=ORIENTED_EDGE('',*,*,#3366,.T.);
#4423=ORIENTED_EDGE('',*,*,#3367,.T.);
#4424=ORIENTED_EDGE('',*,*,#3368,.T.);
#4425=ORIENTED_EDGE('',*,*,#3369,.T.);
#4426=ORIENTED_EDGE('',*,*,#3370,.T.);
#4427=ORIENTED_EDGE('',*,*,#3371,.T.);
#4428=ORIENTED_EDGE('',*,*,#3372,.T.);
#4429=ORIENTED_EDGE('',*,*,#3373,.T.);
#4430=ORIENTED_EDGE('',*,*,#3374,.F.);
#4431=ORIENTED_EDGE('',*,*,#3375,.F.);
#4432=ORIENTED_EDGE('',*,*,#3376,.F.);
#4433=ORIENTED_EDGE('',*,*,#3377,.T.);
#4434=ORIENTED_EDGE('',*,*,#3378,.F.);
#4435=ORIENTED_EDGE('',*,*,#3379,.T.);
#4436=ORIENTED_EDGE('',*,*,#3380,.T.);
#4437=ORIENTED_EDGE('',*,*,#3374,.T.);
#4438=ORIENTED_EDGE('',*,*,#3375,.T.);
#4439=ORIENTED_EDGE('',*,*,#3376,.T.);
#4440=ORIENTED_EDGE('',*,*,#3352,.T.);
#4441=ORIENTED_EDGE('',*,*,#3357,.T.);
#4442=ORIENTED_EDGE('',*,*,#3353,.T.);
#4443=ORIENTED_EDGE('',*,*,#3381,.F.);
#4444=ORIENTED_EDGE('',*,*,#3382,.T.);
#4445=ORIENTED_EDGE('',*,*,#3383,.T.);
#4446=ORIENTED_EDGE('',*,*,#3384,.T.);
#4447=ORIENTED_EDGE('',*,*,#3385,.T.);
#4448=ORIENTED_EDGE('',*,*,#3386,.T.);
#4449=ORIENTED_EDGE('',*,*,#3387,.T.);
#4450=ORIENTED_EDGE('',*,*,#3388,.T.);
#4451=ORIENTED_EDGE('',*,*,#3381,.T.);
#4452=ORIENTED_EDGE('',*,*,#3389,.T.);
#4453=ORIENTED_EDGE('',*,*,#3385,.F.);
#4454=ORIENTED_EDGE('',*,*,#3390,.T.);
#4455=ORIENTED_EDGE('',*,*,#3391,.F.);
#4456=ORIENTED_EDGE('',*,*,#3372,.F.);
#4457=ORIENTED_EDGE('',*,*,#3392,.F.);
#4458=ORIENTED_EDGE('',*,*,#3387,.F.);
#4459=ORIENTED_EDGE('',*,*,#3392,.T.);
#4460=ORIENTED_EDGE('',*,*,#3371,.F.);
#4461=ORIENTED_EDGE('',*,*,#3393,.F.);
#4462=ORIENTED_EDGE('',*,*,#3382,.F.);
#4463=ORIENTED_EDGE('',*,*,#3389,.F.);
#4464=ORIENTED_EDGE('',*,*,#3388,.F.);
#4465=ORIENTED_EDGE('',*,*,#3390,.F.);
#4466=ORIENTED_EDGE('',*,*,#3384,.F.);
#4467=ORIENTED_EDGE('',*,*,#3394,.F.);
#4468=ORIENTED_EDGE('',*,*,#3373,.F.);
#4469=ORIENTED_EDGE('',*,*,#3391,.T.);
#4470=ORIENTED_EDGE('',*,*,#3386,.F.);
#4471=ORIENTED_EDGE('',*,*,#3393,.T.);
#4472=ORIENTED_EDGE('',*,*,#3370,.F.);
#4473=ORIENTED_EDGE('',*,*,#3394,.T.);
#4474=ORIENTED_EDGE('',*,*,#3383,.F.);
#4475=ORIENTED_EDGE('',*,*,#3395,.F.);
#4476=ORIENTED_EDGE('',*,*,#3396,.T.);
#4477=ORIENTED_EDGE('',*,*,#3397,.T.);
#4478=ORIENTED_EDGE('',*,*,#3398,.T.);
#4479=ORIENTED_EDGE('',*,*,#3399,.T.);
#4480=ORIENTED_EDGE('',*,*,#3400,.T.);
#4481=ORIENTED_EDGE('',*,*,#3401,.T.);
#4482=ORIENTED_EDGE('',*,*,#3402,.T.);
#4483=ORIENTED_EDGE('',*,*,#3395,.T.);
#4484=ORIENTED_EDGE('',*,*,#3403,.T.);
#4485=ORIENTED_EDGE('',*,*,#3399,.F.);
#4486=ORIENTED_EDGE('',*,*,#3404,.T.);
#4487=ORIENTED_EDGE('',*,*,#3405,.F.);
#4488=ORIENTED_EDGE('',*,*,#3406,.T.);
#4489=ORIENTED_EDGE('',*,*,#3407,.T.);
#4490=ORIENTED_EDGE('',*,*,#3408,.T.);
#4491=ORIENTED_EDGE('',*,*,#3409,.T.);
#4492=ORIENTED_EDGE('',*,*,#3410,.T.);
#4493=ORIENTED_EDGE('',*,*,#3411,.T.);
#4494=ORIENTED_EDGE('',*,*,#3412,.T.);
#4495=ORIENTED_EDGE('',*,*,#3405,.T.);
#4496=ORIENTED_EDGE('',*,*,#3413,.T.);
#4497=ORIENTED_EDGE('',*,*,#3409,.F.);
#4498=ORIENTED_EDGE('',*,*,#3414,.T.);
#4499=ORIENTED_EDGE('',*,*,#3415,.F.);
#4500=ORIENTED_EDGE('',*,*,#3416,.T.);
#4501=ORIENTED_EDGE('',*,*,#3417,.T.);
#4502=ORIENTED_EDGE('',*,*,#3418,.T.);
#4503=ORIENTED_EDGE('',*,*,#3419,.T.);
#4504=ORIENTED_EDGE('',*,*,#3420,.T.);
#4505=ORIENTED_EDGE('',*,*,#3421,.T.);
#4506=ORIENTED_EDGE('',*,*,#3422,.T.);
#4507=ORIENTED_EDGE('',*,*,#3415,.T.);
#4508=ORIENTED_EDGE('',*,*,#3423,.T.);
#4509=ORIENTED_EDGE('',*,*,#3419,.F.);
#4510=ORIENTED_EDGE('',*,*,#3424,.T.);
#4511=ORIENTED_EDGE('',*,*,#3425,.F.);
#4512=ORIENTED_EDGE('',*,*,#3368,.F.);
#4513=ORIENTED_EDGE('',*,*,#3426,.F.);
#4514=ORIENTED_EDGE('',*,*,#3421,.F.);
#4515=ORIENTED_EDGE('',*,*,#3426,.T.);
#4516=ORIENTED_EDGE('',*,*,#3367,.F.);
#4517=ORIENTED_EDGE('',*,*,#3427,.F.);
#4518=ORIENTED_EDGE('',*,*,#3416,.F.);
#4519=ORIENTED_EDGE('',*,*,#3423,.F.);
#4520=ORIENTED_EDGE('',*,*,#3422,.F.);
#4521=ORIENTED_EDGE('',*,*,#3424,.F.);
#4522=ORIENTED_EDGE('',*,*,#3418,.F.);
#4523=ORIENTED_EDGE('',*,*,#3428,.F.);
#4524=ORIENTED_EDGE('',*,*,#3369,.F.);
#4525=ORIENTED_EDGE('',*,*,#3425,.T.);
#4526=ORIENTED_EDGE('',*,*,#3420,.F.);
#4527=ORIENTED_EDGE('',*,*,#3427,.T.);
#4528=ORIENTED_EDGE('',*,*,#3366,.F.);
#4529=ORIENTED_EDGE('',*,*,#3428,.T.);
#4530=ORIENTED_EDGE('',*,*,#3417,.F.);
#4531=ORIENTED_EDGE('',*,*,#3429,.F.);
#4532=ORIENTED_EDGE('',*,*,#3364,.F.);
#4533=ORIENTED_EDGE('',*,*,#3430,.F.);
#4534=ORIENTED_EDGE('',*,*,#3411,.F.);
#4535=ORIENTED_EDGE('',*,*,#3430,.T.);
#4536=ORIENTED_EDGE('',*,*,#3363,.F.);
#4537=ORIENTED_EDGE('',*,*,#3431,.F.);
#4538=ORIENTED_EDGE('',*,*,#3406,.F.);
#4539=ORIENTED_EDGE('',*,*,#3413,.F.);
#4540=ORIENTED_EDGE('',*,*,#3412,.F.);
#4541=ORIENTED_EDGE('',*,*,#3414,.F.);
#4542=ORIENTED_EDGE('',*,*,#3408,.F.);
#4543=ORIENTED_EDGE('',*,*,#3432,.F.);
#4544=ORIENTED_EDGE('',*,*,#3365,.F.);
#4545=ORIENTED_EDGE('',*,*,#3429,.T.);
#4546=ORIENTED_EDGE('',*,*,#3410,.F.);
#4547=ORIENTED_EDGE('',*,*,#3431,.T.);
#4548=ORIENTED_EDGE('',*,*,#3362,.F.);
#4549=ORIENTED_EDGE('',*,*,#3432,.T.);
#4550=ORIENTED_EDGE('',*,*,#3407,.F.);
#4551=ORIENTED_EDGE('',*,*,#3433,.F.);
#4552=ORIENTED_EDGE('',*,*,#3360,.F.);
#4553=ORIENTED_EDGE('',*,*,#3434,.F.);
#4554=ORIENTED_EDGE('',*,*,#3401,.F.);
#4555=ORIENTED_EDGE('',*,*,#3434,.T.);
#4556=ORIENTED_EDGE('',*,*,#3359,.F.);
#4557=ORIENTED_EDGE('',*,*,#3435,.F.);
#4558=ORIENTED_EDGE('',*,*,#3396,.F.);
#4559=ORIENTED_EDGE('',*,*,#3403,.F.);
#4560=ORIENTED_EDGE('',*,*,#3402,.F.);
#4561=ORIENTED_EDGE('',*,*,#3404,.F.);
#4562=ORIENTED_EDGE('',*,*,#3398,.F.);
#4563=ORIENTED_EDGE('',*,*,#3436,.F.);
#4564=ORIENTED_EDGE('',*,*,#3361,.F.);
#4565=ORIENTED_EDGE('',*,*,#3433,.T.);
#4566=ORIENTED_EDGE('',*,*,#3400,.F.);
#4567=ORIENTED_EDGE('',*,*,#3435,.T.);
#4568=ORIENTED_EDGE('',*,*,#3358,.F.);
#4569=ORIENTED_EDGE('',*,*,#3436,.T.);
#4570=ORIENTED_EDGE('',*,*,#3397,.F.);
#4571=ORIENTED_EDGE('',*,*,#3349,.F.);
#4572=ORIENTED_EDGE('',*,*,#3350,.F.);
#4573=ORIENTED_EDGE('',*,*,#3437,.T.);
#4574=ORIENTED_EDGE('',*,*,#3379,.F.);
#4575=ORIENTED_EDGE('',*,*,#3437,.F.);
#4576=ORIENTED_EDGE('',*,*,#3377,.F.);
#4577=ORIENTED_EDGE('',*,*,#3438,.T.);
#4578=ORIENTED_EDGE('',*,*,#3355,.F.);
#4579=ORIENTED_EDGE('',*,*,#3356,.F.);
#4580=ORIENTED_EDGE('',*,*,#3438,.F.);
#4581=ORIENTED_EDGE('',*,*,#3380,.F.);
#4582=ORIENTED_EDGE('',*,*,#3439,.T.);
#4583=ORIENTED_EDGE('',*,*,#3378,.T.);
#4584=ORIENTED_EDGE('',*,*,#3439,.F.);
#5657=PLANE('',#6422);
#5658=PLANE('',#6425);
#5659=PLANE('',#6431);
#5660=PLANE('',#6433);
#5661=PLANE('',#6442);
#5662=PLANE('',#6444);
#5663=PLANE('',#6449);
#5664=PLANE('',#6451);
#5665=PLANE('',#6456);
#5666=PLANE('',#6458);
#5871=ADVANCED_FACE('',(#822,#654,#655,#656,#657,#658,#659,#660),#513,.T.);
#5872=ADVANCED_FACE('',(#823,#661),#5657,.T.);
#5873=ADVANCED_FACE('',(#824,#662),#5658,.F.);
#5874=ADVANCED_FACE('',(#825),#223,.T.);
#5875=ADVANCED_FACE('',(#826),#224,.T.);
#5876=ADVANCED_FACE('',(#827),#225,.T.);
#5877=ADVANCED_FACE('',(#828),#226,.T.);
#5878=ADVANCED_FACE('',(#829),#514,.T.);
#5879=ADVANCED_FACE('',(#830),#5659,.T.);
#5880=ADVANCED_FACE('',(#831),#5660,.F.);
#5881=ADVANCED_FACE('',(#832),#515,.F.);
#5882=ADVANCED_FACE('',(#833),#209,.F.);
#5883=ADVANCED_FACE('',(#834),#210,.F.);
#5884=ADVANCED_FACE('',(#835),#516,.F.);
#5885=ADVANCED_FACE('',(#836),#517,.T.);
#5886=ADVANCED_FACE('',(#837),#5661,.T.);
#5887=ADVANCED_FACE('',(#838),#5662,.F.);
#5888=ADVANCED_FACE('',(#839),#518,.T.);
#5889=ADVANCED_FACE('',(#840),#5663,.T.);
#5890=ADVANCED_FACE('',(#841),#5664,.F.);
#5891=ADVANCED_FACE('',(#842),#519,.T.);
#5892=ADVANCED_FACE('',(#843),#5665,.T.);
#5893=ADVANCED_FACE('',(#844),#5666,.F.);
#5894=ADVANCED_FACE('',(#845),#520,.F.);
#5895=ADVANCED_FACE('',(#846),#211,.F.);
#5896=ADVANCED_FACE('',(#847),#212,.F.);
#5897=ADVANCED_FACE('',(#848),#521,.F.);
#5898=ADVANCED_FACE('',(#849),#522,.F.);
#5899=ADVANCED_FACE('',(#850),#213,.F.);
#5900=ADVANCED_FACE('',(#851),#214,.F.);
#5901=ADVANCED_FACE('',(#852),#523,.F.);
#5902=ADVANCED_FACE('',(#853),#524,.F.);
#5903=ADVANCED_FACE('',(#854),#215,.F.);
#5904=ADVANCED_FACE('',(#855),#216,.F.);
#5905=ADVANCED_FACE('',(#856),#525,.F.);
#5906=ADVANCED_FACE('',(#857),#217,.T.);
#5907=ADVANCED_FACE('',(#858),#218,.T.);
#5908=ADVANCED_FACE('',(#859),#526,.F.);
#6136=CLOSED_SHELL('',(#5871,#5872,#5873,#5874,#5875,#5876,#5877,#5878,
#5879,#5880,#5881,#5882,#5883,#5884,#5885,#5886,#5887,#5888,#5889,#5890,
#5891,#5892,#5893,#5894,#5895,#5896,#5897,#5898,#5899,#5900,#5901,#5902,
#5903,#5904,#5905,#5906,#5907,#5908));
#6408=AXIS2_PLACEMENT_3D('',#10844,#7292,#7293);
#6409=AXIS2_PLACEMENT_3D('',#10845,#7294,#7295);
#6410=AXIS2_PLACEMENT_3D('',#10848,#7296,#7297);
#6411=AXIS2_PLACEMENT_3D('',#10849,#7298,#7299);
#6412=AXIS2_PLACEMENT_3D('',#10887,#7302,#7303);
#6413=AXIS2_PLACEMENT_3D('',#10888,#7304,#7305);
#6414=AXIS2_PLACEMENT_3D('',#10918,#7307,#7308);
#6415=AXIS2_PLACEMENT_3D('',#10921,#7310,#7311);
#6416=AXIS2_PLACEMENT_3D('',#10926,#7313,#7314);
#6417=AXIS2_PLACEMENT_3D('',#10929,#7316,#7317);
#6418=AXIS2_PLACEMENT_3D('',#10934,#7319,#7320);
#6419=AXIS2_PLACEMENT_3D('',#10937,#7322,#7323);
#6420=AXIS2_PLACEMENT_3D('',#10942,#7325,#7326);
#6421=AXIS2_PLACEMENT_3D('',#10945,#7328,#7329);
#6422=AXIS2_PLACEMENT_3D('',#11081,#7330,#7331);
#6423=AXIS2_PLACEMENT_3D('',#11083,#7332,#7333);
#6424=AXIS2_PLACEMENT_3D('',#11085,#7334,#7335);
#6425=AXIS2_PLACEMENT_3D('',#11086,#7336,#7337);
#6426=AXIS2_PLACEMENT_3D('',#11088,#7338,#7339);
#6427=AXIS2_PLACEMENT_3D('',#11090,#7340,#7341);
#6428=AXIS2_PLACEMENT_3D('',#11151,#7342,#7343);
#6429=AXIS2_PLACEMENT_3D('',#11154,#7344,#7345);
#6430=AXIS2_PLACEMENT_3D('',#11172,#7347,#7348);
#6431=AXIS2_PLACEMENT_3D('',#11188,#7350,#7351);
#6432=AXIS2_PLACEMENT_3D('',#11189,#7352,#7353);
#6433=AXIS2_PLACEMENT_3D('',#11190,#7354,#7355);
#6434=AXIS2_PLACEMENT_3D('',#11191,#7356,#7357);
#6435=AXIS2_PLACEMENT_3D('',#11192,#7358,#7359);
#6436=AXIS2_PLACEMENT_3D('',#11213,#7360,#7361);
#6437=AXIS2_PLACEMENT_3D('',#11224,#7362,#7363);
#6438=AXIS2_PLACEMENT_3D('',#11235,#7364,#7365);
#6439=AXIS2_PLACEMENT_3D('',#11236,#7366,#7367);
#6440=AXIS2_PLACEMENT_3D('',#11239,#7368,#7369);
#6441=AXIS2_PLACEMENT_3D('',#11257,#7371,#7372);
#6442=AXIS2_PLACEMENT_3D('',#11273,#7374,#7375);
#6443=AXIS2_PLACEMENT_3D('',#11274,#7376,#7377);
#6444=AXIS2_PLACEMENT_3D('',#11275,#7378,#7379);
#6445=AXIS2_PLACEMENT_3D('',#11276,#7380,#7381);
#6446=AXIS2_PLACEMENT_3D('',#11277,#7382,#7383);
#6447=AXIS2_PLACEMENT_3D('',#11280,#7384,#7385);
#6448=AXIS2_PLACEMENT_3D('',#11298,#7387,#7388);
#6449=AXIS2_PLACEMENT_3D('',#11314,#7390,#7391);
#6450=AXIS2_PLACEMENT_3D('',#11315,#7392,#7393);
#6451=AXIS2_PLACEMENT_3D('',#11316,#7394,#7395);
#6452=AXIS2_PLACEMENT_3D('',#11317,#7396,#7397);
#6453=AXIS2_PLACEMENT_3D('',#11318,#7398,#7399);
#6454=AXIS2_PLACEMENT_3D('',#11321,#7400,#7401);
#6455=AXIS2_PLACEMENT_3D('',#11339,#7403,#7404);
#6456=AXIS2_PLACEMENT_3D('',#11355,#7406,#7407);
#6457=AXIS2_PLACEMENT_3D('',#11356,#7408,#7409);
#6458=AXIS2_PLACEMENT_3D('',#11357,#7410,#7411);
#6459=AXIS2_PLACEMENT_3D('',#11358,#7412,#7413);
#6460=AXIS2_PLACEMENT_3D('',#11359,#7414,#7415);
#6461=AXIS2_PLACEMENT_3D('',#11380,#7416,#7417);
#6462=AXIS2_PLACEMENT_3D('',#11391,#7418,#7419);
#6463=AXIS2_PLACEMENT_3D('',#11402,#7420,#7421);
#6464=AXIS2_PLACEMENT_3D('',#11403,#7422,#7423);
#6465=AXIS2_PLACEMENT_3D('',#11424,#7424,#7425);
#6466=AXIS2_PLACEMENT_3D('',#11435,#7426,#7427);
#6467=AXIS2_PLACEMENT_3D('',#11446,#7428,#7429);
#6468=AXIS2_PLACEMENT_3D('',#11447,#7430,#7431);
#6469=AXIS2_PLACEMENT_3D('',#11468,#7432,#7433);
#6470=AXIS2_PLACEMENT_3D('',#11479,#7434,#7435);
#6471=AXIS2_PLACEMENT_3D('',#11490,#7436,#7437);
#6472=AXIS2_PLACEMENT_3D('',#11491,#7438,#7439);
#6473=AXIS2_PLACEMENT_3D('',#11492,#7440,#7441);
#6474=AXIS2_PLACEMENT_3D('',#11493,#7442,#7443);
#6475=AXIS2_PLACEMENT_3D('',#11494,#7444,#7445);
#6476=AXIS2_PLACEMENT_3D('',#11495,#7446,#7447);
#7292=DIRECTION('axis',(0.,0.,1.));
#7293=DIRECTION('refdir',(1.,0.,0.));
#7294=DIRECTION('center_axis',(-1.,-1.4811191380744E-16,-1.85154420029064E-16));
#7295=DIRECTION('ref_axis',(-1.85154420029064E-16,0.,1.));
#7296=DIRECTION('center_axis',(1.,1.4811191380744E-16,1.85154420029064E-16));
#7297=DIRECTION('ref_axis',(1.85154420029064E-16,0.,-1.));
#7298=DIRECTION('center_axis',(1.,1.4811191380744E-16,1.85154420029064E-16));
#7299=DIRECTION('ref_axis',(1.85154420029064E-16,0.,-1.));
#7300=DIRECTION('',(1.,1.4811191380744E-16,1.85154420029064E-16));
#7301=DIRECTION('',(1.,1.4811191380744E-16,1.85154420029064E-16));
#7302=DIRECTION('center_axis',(1.,1.4811191380744E-16,1.85154420029064E-16));
#7303=DIRECTION('ref_axis',(1.85154420029064E-16,0.,-1.));
#7304=DIRECTION('center_axis',(1.,1.4811191380744E-16,1.85154420029064E-16));
#7305=DIRECTION('ref_axis',(1.85154420029064E-16,0.,-1.));
#7306=DIRECTION('',(-1.,0.,-1.85037170770859E-16));
#7307=DIRECTION('center_axis',(1.,3.00568153244441E-16,7.87229747683671E-17));
#7308=DIRECTION('ref_axis',(-3.00568153244441E-16,1.,0.));
#7309=DIRECTION('',(-1.,0.,-1.96601993944038E-16));
#7310=DIRECTION('center_axis',(1.,3.00568153244441E-16,7.87229747683671E-17));
#7311=DIRECTION('ref_axis',(-3.00568153244441E-16,1.,0.));
#7312=DIRECTION('',(-1.,0.,0.));
#7313=DIRECTION('center_axis',(1.,4.06999598505139E-16,2.3117921420537E-16));
#7314=DIRECTION('ref_axis',(-4.06999598505139E-16,1.,0.));
#7315=DIRECTION('',(-1.,0.,0.));
#7316=DIRECTION('center_axis',(1.,4.06999598505139E-16,2.3117921420537E-16));
#7317=DIRECTION('ref_axis',(-4.06999598505139E-16,1.,0.));
#7318=DIRECTION('',(-1.,0.,-3.70074341541719E-16));
#7319=DIRECTION('center_axis',(1.,2.54543359068137E-16,3.37610659466067E-16));
#7320=DIRECTION('ref_axis',(3.37610659466067E-16,0.,-1.));
#7321=DIRECTION('',(-1.,0.,-3.70074341541719E-16));
#7322=DIRECTION('center_axis',(1.,2.54543359068137E-16,3.37610659466067E-16));
#7323=DIRECTION('ref_axis',(3.37610659466067E-16,0.,-1.));
#7324=DIRECTION('',(-1.,0.,-1.96601993944038E-16));
#7325=DIRECTION('center_axis',(1.,1.4811191380744E-16,1.85154420029064E-16));
#7326=DIRECTION('ref_axis',(1.85154420029064E-16,0.,-1.));
#7327=DIRECTION('',(-1.,0.,-1.38777878078144E-16));
#7328=DIRECTION('center_axis',(1.,1.4811191380744E-16,1.85154420029064E-16));
#7329=DIRECTION('ref_axis',(1.85154420029064E-16,0.,-1.));
#7330=DIRECTION('center_axis',(1.,1.4811191380744E-16,1.85154420029064E-16));
#7331=DIRECTION('ref_axis',(1.85154420029064E-16,0.,-1.));
#7332=DIRECTION('center_axis',(1.,1.4811191380744E-16,1.85154420029064E-16));
#7333=DIRECTION('ref_axis',(1.85154420029064E-16,0.,-1.));
#7334=DIRECTION('center_axis',(1.,1.4811191380744E-16,1.85154420029064E-16));
#7335=DIRECTION('ref_axis',(1.85154420029064E-16,0.,-1.));
#7336=DIRECTION('center_axis',(1.,1.4811191380744E-16,1.85154420029064E-16));
#7337=DIRECTION('ref_axis',(1.85154420029064E-16,0.,-1.));
#7338=DIRECTION('center_axis',(1.,1.4811191380744E-16,1.85154420029064E-16));
#7339=DIRECTION('ref_axis',(1.85154420029064E-16,0.,-1.));
#7340=DIRECTION('center_axis',(1.,1.4811191380744E-16,1.85154420029064E-16));
#7341=DIRECTION('ref_axis',(1.85154420029064E-16,0.,-1.));
#7342=DIRECTION('center_axis',(-1.,-1.4811191380744E-16,-1.85154420029064E-16));
#7343=DIRECTION('ref_axis',(-1.85154420029064E-16,0.,1.));
#7344=DIRECTION('center_axis',(1.,1.4811191380744E-16,1.85154420029064E-16));
#7345=DIRECTION('ref_axis',(1.85154420029064E-16,0.,-1.));
#7346=DIRECTION('',(-1.,0.,-1.92827419455378E-16));
#7347=DIRECTION('center_axis',(1.,1.4811191380744E-16,1.85154420029064E-16));
#7348=DIRECTION('ref_axis',(1.85154420029064E-16,0.,-1.));
#7349=DIRECTION('',(-1.,0.,-1.65280645247467E-16));
#7350=DIRECTION('center_axis',(1.,1.4811191380744E-16,1.85154420029064E-16));
#7351=DIRECTION('ref_axis',(1.85154420029064E-16,0.,-1.));
#7352=DIRECTION('center_axis',(1.,1.4811191380744E-16,1.85154420029064E-16));
#7353=DIRECTION('ref_axis',(1.85154420029064E-16,0.,-1.));
#7354=DIRECTION('center_axis',(1.,1.4811191380744E-16,1.85154420029064E-16));
#7355=DIRECTION('ref_axis',(1.85154420029064E-16,0.,-1.));
#7356=DIRECTION('center_axis',(1.,1.4811191380744E-16,1.85154420029064E-16));
#7357=DIRECTION('ref_axis',(1.85154420029064E-16,0.,-1.));
#7358=DIRECTION('center_axis',(1.,1.4811191380744E-16,1.85154420029064E-16));
#7359=DIRECTION('ref_axis',(1.85154420029064E-16,0.,-1.));
#7360=DIRECTION('center_axis',(1.,1.4811191380744E-16,1.85154420029064E-16));
#7361=DIRECTION('ref_axis',(3.15796771448933E-16,0.,-1.));
#7362=DIRECTION('center_axis',(1.,1.4811191380744E-16,1.85154420029064E-16));
#7363=DIRECTION('ref_axis',(3.15796771448933E-16,0.,-1.));
#7364=DIRECTION('center_axis',(1.,1.4811191380744E-16,1.85154420029064E-16));
#7365=DIRECTION('ref_axis',(1.85154420029064E-16,0.,-1.));
#7366=DIRECTION('center_axis',(-1.,-3.00568153244441E-16,-7.87229747683671E-17));
#7367=DIRECTION('ref_axis',(3.00568153244441E-16,-1.,0.));
#7368=DIRECTION('center_axis',(1.,3.00568153244441E-16,7.87229747683671E-17));
#7369=DIRECTION('ref_axis',(-3.0056815324444E-16,1.,-1.04744440165294E-14));
#7370=DIRECTION('',(-1.,0.,-5.50935484158224E-17));
#7371=DIRECTION('center_axis',(1.,3.00568153244441E-16,7.87229747683671E-17));
#7372=DIRECTION('ref_axis',(-3.0056815324444E-16,1.,-1.04744440165294E-14));
#7373=DIRECTION('',(-1.,0.,-8.26403226237337E-17));
#7374=DIRECTION('center_axis',(1.,3.00568153244441E-16,7.87229747683671E-17));
#7375=DIRECTION('ref_axis',(7.87229747683671E-17,0.,-1.));
#7376=DIRECTION('center_axis',(1.,3.00568153244441E-16,7.87229747683671E-17));
#7377=DIRECTION('ref_axis',(-3.00568153244441E-16,1.,0.));
#7378=DIRECTION('center_axis',(1.,3.00568153244441E-16,7.87229747683671E-17));
#7379=DIRECTION('ref_axis',(7.87229747683671E-17,0.,-1.));
#7380=DIRECTION('center_axis',(1.,3.00568153244441E-16,7.87229747683671E-17));
#7381=DIRECTION('ref_axis',(-3.00568153244441E-16,1.,0.));
#7382=DIRECTION('center_axis',(-1.,-4.06999598505139E-16,-2.3117921420537E-16));
#7383=DIRECTION('ref_axis',(4.06999598505139E-16,-1.,0.));
#7384=DIRECTION('center_axis',(1.,4.06999598505139E-16,2.3117921420537E-16));
#7385=DIRECTION('ref_axis',(-2.3117921420537E-16,-1.27744465495421E-32,
1.));
#7386=DIRECTION('',(-1.,-4.4074838732658E-16,-4.4074838732658E-16));
#7387=DIRECTION('center_axis',(1.,4.06999598505139E-16,2.3117921420537E-16));
#7388=DIRECTION('ref_axis',(-2.3117921420537E-16,-1.27744465495421E-32,
1.));
#7389=DIRECTION('',(-1.,-8.81496774653158E-16,-4.40748387326579E-16));
#7390=DIRECTION('center_axis',(1.,4.06999598505139E-16,2.3117921420537E-16));
#7391=DIRECTION('ref_axis',(2.3117921420537E-16,0.,-1.));
#7392=DIRECTION('center_axis',(1.,4.06999598505139E-16,2.3117921420537E-16));
#7393=DIRECTION('ref_axis',(-4.06999598505139E-16,1.,0.));
#7394=DIRECTION('center_axis',(1.,4.06999598505139E-16,2.3117921420537E-16));
#7395=DIRECTION('ref_axis',(2.3117921420537E-16,0.,-1.));
#7396=DIRECTION('center_axis',(1.,4.06999598505139E-16,2.3117921420537E-16));
#7397=DIRECTION('ref_axis',(-4.06999598505139E-16,1.,0.));
#7398=DIRECTION('center_axis',(-1.,-2.54543359068137E-16,-3.37610659466067E-16));
#7399=DIRECTION('ref_axis',(5.87374514062376E-17,0.707106781186545,-0.70710678118655));
#7400=DIRECTION('center_axis',(1.,2.54543359068137E-16,3.37610659466067E-16));
#7401=DIRECTION('ref_axis',(2.54543359068136E-16,-1.,3.49148133884313E-15));
#7402=DIRECTION('',(-1.,0.,0.));
#7403=DIRECTION('center_axis',(1.,2.54543359068137E-16,3.37610659466067E-16));
#7404=DIRECTION('ref_axis',(2.54543359068136E-16,-1.,3.49148133884313E-15));
#7405=DIRECTION('',(-1.,0.,-4.40748387326579E-16));
#7406=DIRECTION('center_axis',(1.,2.54543359068137E-16,3.37610659466067E-16));
#7407=DIRECTION('ref_axis',(3.37610659466067E-16,0.,-1.));
#7408=DIRECTION('center_axis',(1.,2.54543359068137E-16,3.37610659466067E-16));
#7409=DIRECTION('ref_axis',(3.37610659466067E-16,0.,-1.));
#7410=DIRECTION('center_axis',(1.,2.54543359068137E-16,3.37610659466067E-16));
#7411=DIRECTION('ref_axis',(3.37610659466067E-16,0.,-1.));
#7412=DIRECTION('center_axis',(1.,2.54543359068137E-16,3.37610659466067E-16));
#7413=DIRECTION('ref_axis',(3.37610659466067E-16,0.,-1.));
#7414=DIRECTION('center_axis',(1.,1.4811191380744E-16,1.85154420029064E-16));
#7415=DIRECTION('ref_axis',(1.85154420029064E-16,0.,-1.));
#7416=DIRECTION('center_axis',(1.,2.54543359068137E-16,3.37610659466067E-16));
#7417=DIRECTION('ref_axis',(3.15796771448933E-16,0.,-1.));
#7418=DIRECTION('center_axis',(1.,2.54543359068137E-16,3.37610659466067E-16));
#7419=DIRECTION('ref_axis',(3.15796771448933E-16,0.,-1.));
#7420=DIRECTION('center_axis',(1.,2.54543359068137E-16,3.37610659466067E-16));
#7421=DIRECTION('ref_axis',(-3.22551558256129E-16,-0.0570045103629633,0.99837392083241));
#7422=DIRECTION('center_axis',(1.,1.4811191380744E-16,1.85154420029064E-16));
#7423=DIRECTION('ref_axis',(-1.93296391409384E-16,0.0570045103629774,0.998373920832409));
#7424=DIRECTION('center_axis',(1.,4.06999598505139E-16,2.3117921420537E-16));
#7425=DIRECTION('ref_axis',(3.15796771448933E-16,0.,-1.));
#7426=DIRECTION('center_axis',(1.,4.06999598505139E-16,2.3117921420537E-16));
#7427=DIRECTION('ref_axis',(3.15796771448933E-16,0.,-1.));
#7428=DIRECTION('center_axis',(1.,4.06999598505139E-16,2.3117921420537E-16));
#7429=DIRECTION('ref_axis',(-4.06999598505139E-16,1.,0.));
#7430=DIRECTION('center_axis',(1.,1.4811191380744E-16,1.85154420029064E-16));
#7431=DIRECTION('ref_axis',(1.85154420029064E-16,0.,-1.));
#7432=DIRECTION('center_axis',(1.,3.00568153244441E-16,7.87229747683671E-17));
#7433=DIRECTION('ref_axis',(0.,0.,-1.));
#7434=DIRECTION('center_axis',(1.,3.00568153244441E-16,7.87229747683671E-17));
#7435=DIRECTION('ref_axis',(0.,0.,-1.));
#7436=DIRECTION('center_axis',(1.,3.00568153244441E-16,7.87229747683671E-17));
#7437=DIRECTION('ref_axis',(-3.00568153244441E-16,1.,0.));
#7438=DIRECTION('center_axis',(1.,1.4811191380744E-16,1.85154420029064E-16));
#7439=DIRECTION('ref_axis',(3.46606212565903E-16,0.,-1.));
#7440=DIRECTION('center_axis',(1.4811191380744E-16,-1.,3.20853184254275E-32));
#7441=DIRECTION('ref_axis',(-2.16628882853689E-16,0.,1.));
#7442=DIRECTION('center_axis',(1.,1.4811191380744E-16,1.85154420029064E-16));
#7443=DIRECTION('ref_axis',(3.46606212565902E-16,0.,-1.));
#7444=DIRECTION('center_axis',(1.4811191380744E-16,-1.,0.));
#7445=DIRECTION('ref_axis',(0.,0.,1.));
#7446=DIRECTION('center_axis',(1.,1.4811191380744E-16,1.85154420029064E-16));
#7447=DIRECTION('ref_axis',(1.85154420029064E-16,0.,-1.));
#7448=DIRECTION('',(1.,1.4811191380744E-16,1.85154420029064E-16));
#10844=CARTESIAN_POINT('',(0.,0.,0.));
#10845=CARTESIAN_POINT('Origin',(50.,54.6122755947453,-11.9999999999999));
#10846=CARTESIAN_POINT('',(36.,54.6122755947453,-32.4999999999999));
#10847=CARTESIAN_POINT('',(36.,54.6122755947453,8.50000000000008));
#10848=CARTESIAN_POINT('Origin',(36.,54.6122755947453,-11.9999999999999));
#10849=CARTESIAN_POINT('Origin',(36.,54.6122755947453,-11.9999999999999));
#10850=CARTESIAN_POINT('',(36.603289189263,54.6122755947453,-32.4999999999999));
#10851=CARTESIAN_POINT('',(50.,54.6122755947453,-32.4999999999999));
#10852=CARTESIAN_POINT('',(36.7497490222913,54.2658144588871,-32.4970721002132));
#10853=CARTESIAN_POINT('Ctrl Pts',(36.7497490222914,54.2658144588871,-32.4970721002132));
#10854=CARTESIAN_POINT('Ctrl Pts',(36.7079677621958,54.3157388332819,-32.4979159697851));
#10855=CARTESIAN_POINT('Ctrl Pts',(36.6713203406449,54.3700115492414,-32.4986487617911));
#10856=CARTESIAN_POINT('Ctrl Pts',(36.6219970312668,54.4788517884076,-32.4996303938589));
#10857=CARTESIAN_POINT('Ctrl Pts',(36.6075439138862,54.5320464525539,-32.4999158675413));
#10858=CARTESIAN_POINT('Ctrl Pts',(36.6035546196614,54.5952824394035,-32.4999947523746));
#10859=CARTESIAN_POINT('Ctrl Pts',(36.6032891892631,54.6038064661215,-32.4999999999999));
#10860=CARTESIAN_POINT('Ctrl Pts',(36.6032891892631,54.6122755947453,-32.4999999999999));
#10861=CARTESIAN_POINT('',(48.396710810737,54.6122755947453,-32.4999999999999));
#10862=CARTESIAN_POINT('Ctrl Pts',(48.396710810737,54.6122755947453,-32.4999999999999));
#10863=CARTESIAN_POINT('Ctrl Pts',(48.396710810737,54.5998907719614,-32.4999999999999));
#10864=CARTESIAN_POINT('Ctrl Pts',(48.3961431217452,54.5874935361619,-32.4999887774468));
#10865=CARTESIAN_POINT('Ctrl Pts',(48.3891968128691,54.5117737928711,-32.4998514003519));
#10866=CARTESIAN_POINT('Ctrl Pts',(48.3690498018801,54.4529115279532,-32.4994531179785));
#10867=CARTESIAN_POINT('Ctrl Pts',(48.2945766533058,54.3105701888654,-32.49796779174));
#10868=CARTESIAN_POINT('Ctrl Pts',(48.224634010684,54.229506699135,-32.4965615873769));
#10869=CARTESIAN_POINT('Ctrl Pts',(47.9894682579553,54.0138621012104,-32.4917505532513));
#10870=CARTESIAN_POINT('Ctrl Pts',(47.790194476128,53.8921934273276,-32.4875698440548));
#10871=CARTESIAN_POINT('Ctrl Pts',(47.2591893370102,53.6095844257818,-32.4763245946928));
#10872=CARTESIAN_POINT('Ctrl Pts',(46.8036941106391,53.4296399345416,-32.4664417842137));
#10873=CARTESIAN_POINT('Ctrl Pts',(44.8908589619487,52.8583430003526,-32.4291083452159));
#10874=CARTESIAN_POINT('Ctrl Pts',(43.0234357271856,52.6236088262441,-32.4042961436254));
#10875=CARTESIAN_POINT('Ctrl Pts',(39.8390803845175,52.9459866017737,-32.4325402594283));
#10876=CARTESIAN_POINT('Ctrl Pts',(38.8321900018614,53.205505452804,-32.4535208321079));
#10877=CARTESIAN_POINT('Ctrl Pts',(37.7302514044692,53.6201478825653,-32.476460031332));
#10878=CARTESIAN_POINT('Ctrl Pts',(37.4193174431745,53.768280734008,-32.483158770581));
#10879=CARTESIAN_POINT('Ctrl Pts',(37.0379364071817,54.0043124559943,-32.4911694687953));
#10880=CARTESIAN_POINT('Ctrl Pts',(36.8894774405333,54.1120017210872,-32.4942401368472));
#10881=CARTESIAN_POINT('Ctrl Pts',(36.7699059821373,54.2423162108141,-32.4966645914004));
#10882=CARTESIAN_POINT('Ctrl Pts',(36.7596837012345,54.25394352369,-32.4968714463016));
#10883=CARTESIAN_POINT('Ctrl Pts',(36.7497490222914,54.2658144588871,-32.4970721002132));
#10884=CARTESIAN_POINT('',(49.,54.6122755947453,-32.4999999999999));
#10885=CARTESIAN_POINT('',(50.,54.6122755947453,-32.4999999999999));
#10886=CARTESIAN_POINT('',(49.,54.6122755947453,8.50000000000009));
#10887=CARTESIAN_POINT('Origin',(49.,54.6122755947453,-11.9999999999999));
#10888=CARTESIAN_POINT('Origin',(49.,54.6122755947453,-11.9999999999999));
#10889=CARTESIAN_POINT('Ctrl Pts',(36.603289189263,54.6122755947453,-32.4999999999999));
#10890=CARTESIAN_POINT('Ctrl Pts',(36.603289189263,54.6608249084485,-32.4999999999999));
#10891=CARTESIAN_POINT('Ctrl Pts',(36.6119924398781,54.7075701848921,-32.4998281802077));
#10892=CARTESIAN_POINT('Ctrl Pts',(36.6545156775753,54.8307810795885,-32.4989841905835));
#10893=CARTESIAN_POINT('Ctrl Pts',(36.7008380045797,54.9008048487387,-32.4980603157128));
#10894=CARTESIAN_POINT('Ctrl Pts',(36.8625317111402,55.0923640981108,-32.4947934283504));
#10895=CARTESIAN_POINT('Ctrl Pts',(37.0198338309866,55.2093236387767,-32.4915503477017));
#10896=CARTESIAN_POINT('Ctrl Pts',(37.4320685633155,55.4637121723344,-32.482889935361));
#10897=CARTESIAN_POINT('Ctrl Pts',(37.7488381293379,55.611880231403,-32.4760684685696));
#10898=CARTESIAN_POINT('Ctrl Pts',(39.1601676320809,56.1410407225304,-32.4467069002989));
#10899=CARTESIAN_POINT('Ctrl Pts',(40.717083195287,56.4741768433207,-32.4152718262714));
#10900=CARTESIAN_POINT('Ctrl Pts',(42.5,56.4741768433207,-32.4152718262714));
#10901=CARTESIAN_POINT('Ctrl Pts',(43.4574590376155,56.4741768433207,-32.4152718262714));
#10902=CARTESIAN_POINT('Ctrl Pts',(44.4269153217986,56.3794041517536,-32.4246324531227));
#10903=CARTESIAN_POINT('Ctrl Pts',(46.1871857836264,56.0096519365651,-32.4530673729712));
#10904=CARTESIAN_POINT('Ctrl Pts',(46.8757138664064,55.7779082090869,-32.4681777143441));
#10905=CARTESIAN_POINT('Ctrl Pts',(47.6009912659702,55.4395958991355,-32.4835638316369));
#10906=CARTESIAN_POINT('Ctrl Pts',(47.8399918525533,55.309998820274,-32.4886343233478));
#10907=CARTESIAN_POINT('Ctrl Pts',(48.1243771925797,55.091934993814,-32.4945190874943));
#10908=CARTESIAN_POINT('Ctrl Pts',(48.2195690308988,55.0050263124739,-32.4964575266732));
#10909=CARTESIAN_POINT('Ctrl Pts',(48.3274797628088,54.8557541081654,-32.4986259493983));
#10910=CARTESIAN_POINT('Ctrl Pts',(48.3595242538026,54.796889883988,-32.4992631372541));
#10911=CARTESIAN_POINT('Ctrl Pts',(48.3905089403897,54.6939813738137,-32.4998775530034));
#10912=CARTESIAN_POINT('Ctrl Pts',(48.396710810737,54.6531962409273,-32.4999999999999));
#10913=CARTESIAN_POINT('Ctrl Pts',(48.396710810737,54.6122755947453,-32.4999999999999));
#10914=CARTESIAN_POINT('',(36.5,41.5141044679107,3.76984188672031));
#10915=CARTESIAN_POINT('',(48.5,41.5141044679107,3.76984188672031));
#10916=CARTESIAN_POINT('',(48.5,41.5141044679107,3.76984188672031));
#10917=CARTESIAN_POINT('',(48.5,38.8424337080254,1.09817112683513));
#10918=CARTESIAN_POINT('Origin',(48.5,54.6122755947453,-11.9999999999999));
#10919=CARTESIAN_POINT('',(36.5,38.8424337080254,1.09817112683513));
#10920=CARTESIAN_POINT('',(48.5,38.8424337080254,1.09817112683513));
#10921=CARTESIAN_POINT('Origin',(36.5,54.6122755947453,-11.9999999999999));
#10922=CARTESIAN_POINT('',(36.5,38.8424337080252,-25.0981711268347));
#10923=CARTESIAN_POINT('',(48.5,38.8424337080252,-25.0981711268347));
#10924=CARTESIAN_POINT('',(48.5,38.8424337080252,-25.0981711268347));
#10925=CARTESIAN_POINT('',(48.5,41.5141044679105,-27.7698418867199));
#10926=CARTESIAN_POINT('Origin',(48.5,54.6122755947453,-11.9999999999999));
#10927=CARTESIAN_POINT('',(36.5,41.5141044679105,-27.7698418867199));
#10928=CARTESIAN_POINT('',(48.5,41.5141044679105,-27.7698418867199));
#10929=CARTESIAN_POINT('Origin',(36.5,54.6122755947453,-11.9999999999999));
#10930=CARTESIAN_POINT('',(36.5,67.7104467215801,-27.7698418867201));
#10931=CARTESIAN_POINT('',(48.5,67.7104467215801,-27.7698418867201));
#10932=CARTESIAN_POINT('',(48.5,67.7104467215801,-27.7698418867201));
#10933=CARTESIAN_POINT('',(48.5,70.3821174814653,-25.0981711268349));
#10934=CARTESIAN_POINT('Origin',(48.5,54.6122755947453,-11.9999999999999));
#10935=CARTESIAN_POINT('',(36.5,70.3821174814653,-25.0981711268349));
#10936=CARTESIAN_POINT('',(48.5,70.3821174814653,-25.0981711268349));
#10937=CARTESIAN_POINT('Origin',(36.5,54.6122755947453,-11.9999999999999));
#10938=CARTESIAN_POINT('',(36.5,70.3821174814654,1.09817112683487));
#10939=CARTESIAN_POINT('',(48.5,70.3821174814654,1.09817112683488));
#10940=CARTESIAN_POINT('',(48.5,70.3821174814654,1.09817112683488));
#10941=CARTESIAN_POINT('',(48.5,67.7104467215802,3.76984188672011));
#10942=CARTESIAN_POINT('Origin',(48.5,54.6122755947453,-11.9999999999999));
#10943=CARTESIAN_POINT('',(36.5,67.7104467215802,3.76984188672011));
#10944=CARTESIAN_POINT('',(48.5,67.7104467215802,3.76984188672011));
#10945=CARTESIAN_POINT('Origin',(36.5,54.6122755947453,-11.9999999999999));
#10946=CARTESIAN_POINT('',(36.7497652551312,75.1093469933142,-12.3464475251848));
#10947=CARTESIAN_POINT('Ctrl Pts',(42.5,75.0275474210168,-13.8619012485751));
#10948=CARTESIAN_POINT('Ctrl Pts',(41.5425409623847,75.0275474210168,-13.8619012485751));
#10949=CARTESIAN_POINT('Ctrl Pts',(40.5730846782014,75.0369080478681,-13.767128557008));
#10950=CARTESIAN_POINT('Ctrl Pts',(38.8128142163727,75.0653429677166,-13.3973763418193));
#10951=CARTESIAN_POINT('Ctrl Pts',(38.124286133593,75.0804533090896,-13.165632614341));
#10952=CARTESIAN_POINT('Ctrl Pts',(37.39900873403,75.0958394263824,-12.82732030439));
#10953=CARTESIAN_POINT('Ctrl Pts',(37.1600081474468,75.1009099180932,-12.6977232255284));
#10954=CARTESIAN_POINT('Ctrl Pts',(36.8756228074202,75.1067946822398,-12.4796593990683));
#10955=CARTESIAN_POINT('Ctrl Pts',(36.7804309691012,75.1087331214186,-12.3927507177283));
#10956=CARTESIAN_POINT('Ctrl Pts',(36.6725202371911,75.1109015441437,-12.2434785134197));
#10957=CARTESIAN_POINT('Ctrl Pts',(36.6404757461974,75.1115387319995,-12.1846142892423));
#10958=CARTESIAN_POINT('Ctrl Pts',(36.60578337376,75.1122266698925,-12.0693915532655));
#10959=CARTESIAN_POINT('Ctrl Pts',(36.6000950949635,75.1123387689502,-12.0162240743446));
#10960=CARTESIAN_POINT('Ctrl Pts',(36.6108031871309,75.1121269950974,-11.8994981981255));
#10961=CARTESIAN_POINT('Ctrl Pts',(36.63095019812,75.1117287127239,-11.8406359332075));
#10962=CARTESIAN_POINT('Ctrl Pts',(36.705423346694,75.1102433864854,-11.6982945941202));
#10963=CARTESIAN_POINT('Ctrl Pts',(36.7753659893155,75.1088371821223,-11.6172311043898));
#10964=CARTESIAN_POINT('Ctrl Pts',(37.0105317420447,75.1040261479967,-11.4015865064648));
#10965=CARTESIAN_POINT('Ctrl Pts',(37.2098055238719,75.0998454388001,-11.279917832582));
#10966=CARTESIAN_POINT('Ctrl Pts',(37.7408106629901,75.0886001894382,-10.997308831036));
#10967=CARTESIAN_POINT('Ctrl Pts',(38.1963058893614,75.0787173789591,-10.8173643397959));
#10968=CARTESIAN_POINT('Ctrl Pts',(40.1091410380511,75.0413839399612,-10.2460674056071));
#10969=CARTESIAN_POINT('Ctrl Pts',(41.9765642728142,75.0165717383708,-10.0113332314985));
#10970=CARTESIAN_POINT('Ctrl Pts',(45.1609196154824,75.0448158541737,-10.3337110070281));
#10971=CARTESIAN_POINT('Ctrl Pts',(46.1678099981386,75.0657964268533,-10.5932298580583));
#10972=CARTESIAN_POINT('Ctrl Pts',(47.2697485955313,75.0887356260774,-11.0078722878199));
#10973=CARTESIAN_POINT('Ctrl Pts',(47.5806825568259,75.0954343653265,-11.1560051392625));
#10974=CARTESIAN_POINT('Ctrl Pts',(47.9620635928186,75.1034450635407,-11.3920368612488));
#10975=CARTESIAN_POINT('Ctrl Pts',(48.1105225594667,75.1065157315926,-11.4997261263416));
#10976=CARTESIAN_POINT('Ctrl Pts',(48.2739688645561,75.10982980122,-11.6778574474043));
#10977=CARTESIAN_POINT('Ctrl Pts',(48.3224965288387,75.1108012999275,-11.7440918293815));
#10978=CARTESIAN_POINT('Ctrl Pts',(48.3780029687331,75.1119059886043,-11.8665761936618));
#10979=CARTESIAN_POINT('Ctrl Pts',(48.3924560861139,75.1121914622867,-11.9197708578082));
#10980=CARTESIAN_POINT('Ctrl Pts',(48.3995482155258,75.1123317029947,-12.0321911950802));
#10981=CARTESIAN_POINT('Ctrl Pts',(48.3907243897671,75.112157697847,-12.0874225881673));
#10982=CARTESIAN_POINT('Ctrl Pts',(48.3454843224248,75.111259785329,-12.2185054848428));
#10983=CARTESIAN_POINT('Ctrl Pts',(48.2991619954204,75.1103359104582,-12.2885292539931));
#10984=CARTESIAN_POINT('Ctrl Pts',(48.1374682888594,75.1070690230958,-12.4800885033658));
#10985=CARTESIAN_POINT('Ctrl Pts',(47.9801661690123,75.1038259424471,-12.5970480440319));
#10986=CARTESIAN_POINT('Ctrl Pts',(47.567931436684,75.0951655301064,-12.8514365775891));
#10987=CARTESIAN_POINT('Ctrl Pts',(47.2511618706613,75.088344063315,-12.9996046366577));
#10988=CARTESIAN_POINT('Ctrl Pts',(45.8398323679192,75.0589824950443,-13.5287651277848));
#10989=CARTESIAN_POINT('Ctrl Pts',(44.2829168047132,75.0275474210168,-13.8619012485751));
#10990=CARTESIAN_POINT('Ctrl Pts',(42.5,75.0275474210168,-13.8619012485751));
#10991=CARTESIAN_POINT('',(36.7497162970046,54.2657870626157,8.49707235020499));
#10992=CARTESIAN_POINT('Ctrl Pts',(42.5,56.4741768433204,8.41527182627157));
#10993=CARTESIAN_POINT('Ctrl Pts',(41.5425409623847,56.4741768433204,8.41527182627157));
#10994=CARTESIAN_POINT('Ctrl Pts',(40.5730846782016,56.3794041517534,8.42463245312286));
#10995=CARTESIAN_POINT('Ctrl Pts',(38.8128142163725,56.0096519365646,8.45306737297136));
#10996=CARTESIAN_POINT('Ctrl Pts',(38.1242861335929,55.7779082090862,8.46817771434433));
#10997=CARTESIAN_POINT('Ctrl Pts',(37.3990087340298,55.4395958991352,8.48356383163711));
#10998=CARTESIAN_POINT('Ctrl Pts',(37.1600081474467,55.3099988202737,8.48863432334797));
#10999=CARTESIAN_POINT('Ctrl Pts',(36.8756228074202,55.0919349938136,8.49451908749452));
#11000=CARTESIAN_POINT('Ctrl Pts',(36.7804309691012,55.0050263124736,8.49645752667339));
#11001=CARTESIAN_POINT('Ctrl Pts',(36.6725202371913,54.8557541081652,8.49862594939842));
#11002=CARTESIAN_POINT('Ctrl Pts',(36.6404757461974,54.7968898839877,8.49926313725424));
#11003=CARTESIAN_POINT('Ctrl Pts',(36.60578337376,54.6816671480108,8.4999510751473));
#11004=CARTESIAN_POINT('Ctrl Pts',(36.6000950949635,54.6284996690899,8.50006317420492));
#11005=CARTESIAN_POINT('Ctrl Pts',(36.6108031871309,54.5117737928708,8.4998514003521));
#11006=CARTESIAN_POINT('Ctrl Pts',(36.63095019812,54.4529115279528,8.49945311797868));
#11007=CARTESIAN_POINT('Ctrl Pts',(36.7054233466942,54.3105701888652,8.49796779174013));
#11008=CARTESIAN_POINT('Ctrl Pts',(36.7753659893159,54.2295066991348,8.49656158737708));
#11009=CARTESIAN_POINT('Ctrl Pts',(37.0105317420448,54.01386210121,8.49175055325143));
#11010=CARTESIAN_POINT('Ctrl Pts',(37.2098055238722,53.8921934273273,8.48756984405489));
#11011=CARTESIAN_POINT('Ctrl Pts',(37.7408106629893,53.6095844257818,8.47632459469298));
#11012=CARTESIAN_POINT('Ctrl Pts',(38.1963058893602,53.4296399345416,8.46644178421388));
#11013=CARTESIAN_POINT('Ctrl Pts',(40.1091410380517,52.8583430003522,8.42910834521598));
#11014=CARTESIAN_POINT('Ctrl Pts',(41.9765642728151,52.623608826244,8.40429614362558));
#11015=CARTESIAN_POINT('Ctrl Pts',(45.1609196154835,52.9459866017735,8.43254025942847));
#11016=CARTESIAN_POINT('Ctrl Pts',(46.1678099981393,53.2055054528039,8.45352083210801));
#11017=CARTESIAN_POINT('Ctrl Pts',(47.2697485955285,53.6201478825642,8.47646003133207));
#11018=CARTESIAN_POINT('Ctrl Pts',(47.5806825568242,53.7682807340069,8.48315877058117));
#11019=CARTESIAN_POINT('Ctrl Pts',(47.9620635928186,54.0043124559941,8.49116946879544));
#11020=CARTESIAN_POINT('Ctrl Pts',(48.1105225594668,54.112001721087,8.49424013684733));
#11021=CARTESIAN_POINT('Ctrl Pts',(48.2739688645561,54.2901330421496,8.49755420647477));
#11022=CARTESIAN_POINT('Ctrl Pts',(48.3224965288387,54.3563674241268,8.49852570518227));
#11023=CARTESIAN_POINT('Ctrl Pts',(48.3780029687332,54.4788517884074,8.49963039385909));
#11024=CARTESIAN_POINT('Ctrl Pts',(48.3924560861139,54.5320464525537,8.49991586754141));
#11025=CARTESIAN_POINT('Ctrl Pts',(48.3995482155258,54.6444667898256,8.50005610824948));
#11026=CARTESIAN_POINT('Ctrl Pts',(48.390724389767,54.6996981829127,8.49988210310169));
#11027=CARTESIAN_POINT('Ctrl Pts',(48.3454843224248,54.8307810795882,8.49898419058371));
#11028=CARTESIAN_POINT('Ctrl Pts',(48.2991619954204,54.9008048487383,8.498060315713));
#11029=CARTESIAN_POINT('Ctrl Pts',(48.13746828886,55.0923640981104,8.49479342835062));
#11030=CARTESIAN_POINT('Ctrl Pts',(47.9801661690137,55.2093236387763,8.49155034770193));
#11031=CARTESIAN_POINT('Ctrl Pts',(47.5679314366844,55.4637121723342,8.48288993536117));
#11032=CARTESIAN_POINT('Ctrl Pts',(47.251161870662,55.6118802314028,8.47606846856981));
#11033=CARTESIAN_POINT('Ctrl Pts',(45.8398323679184,56.1410407225304,8.4467069002991));
#11034=CARTESIAN_POINT('Ctrl Pts',(44.2829168047119,56.4741768433204,8.41527182627157));
#11035=CARTESIAN_POINT('Ctrl Pts',(42.5,56.4741768433204,8.41527182627157));
#11036=CARTESIAN_POINT('',(36.7497162970046,34.1152032445404,-12.3464885321295));
#11037=CARTESIAN_POINT('Ctrl Pts',(42.5,34.1970037684738,-10.1380987514247));
#11038=CARTESIAN_POINT('Ctrl Pts',(41.5425409623847,34.1970037684738,-10.1380987514247));
#11039=CARTESIAN_POINT('Ctrl Pts',(40.5730846782015,34.1876431416225,-10.2328714429918));
#11040=CARTESIAN_POINT('Ctrl Pts',(38.8128142163735,34.1592082217741,-10.6026236581803));
#11041=CARTESIAN_POINT('Ctrl Pts',(38.1242861335935,34.1440978804011,-10.8343673856586));
#11042=CARTESIAN_POINT('Ctrl Pts',(37.39900873403,34.1287117631083,-11.1726796956099));
#11043=CARTESIAN_POINT('Ctrl Pts',(37.1600081474469,34.1236412713974,-11.3022767744714));
#11044=CARTESIAN_POINT('Ctrl Pts',(36.8756228074203,34.1177565072509,-11.5203406009315));
#11045=CARTESIAN_POINT('Ctrl Pts',(36.7804309691013,34.115818068072,-11.6072492822715));
#11046=CARTESIAN_POINT('Ctrl Pts',(36.6725202371913,34.113649645347,-11.75652148658));
#11047=CARTESIAN_POINT('Ctrl Pts',(36.6404757461974,34.1130124574912,-11.8153857107575));
#11048=CARTESIAN_POINT('Ctrl Pts',(36.60578337376,34.1123245195981,-11.9306084467343));
#11049=CARTESIAN_POINT('Ctrl Pts',(36.6000950949635,34.1122124205405,-11.9837759256552));
#11050=CARTESIAN_POINT('Ctrl Pts',(36.6108031871309,34.1124241943933,-12.1005018018743));
#11051=CARTESIAN_POINT('Ctrl Pts',(36.63095019812,34.1128224767667,-12.1593640667924));
#11052=CARTESIAN_POINT('Ctrl Pts',(36.7054233466949,34.1143078030053,-12.3017054058813));
#11053=CARTESIAN_POINT('Ctrl Pts',(36.7753659893176,34.1157140073684,-12.3827688956119));
#11054=CARTESIAN_POINT('Ctrl Pts',(37.0105317420447,34.120525041494,-12.598413493535));
#11055=CARTESIAN_POINT('Ctrl Pts',(37.2098055238719,34.1247057506905,-12.7200821674178));
#11056=CARTESIAN_POINT('Ctrl Pts',(37.7408106629894,34.1359510000524,-13.0026911689634));
#11057=CARTESIAN_POINT('Ctrl Pts',(38.1963058893603,34.1458338105315,-13.1826356602036));
#11058=CARTESIAN_POINT('Ctrl Pts',(40.1091410380501,34.1831672495294,-13.7539325943925));
#11059=CARTESIAN_POINT('Ctrl Pts',(41.9765642728128,34.2079794511198,-13.9886667685015));
#11060=CARTESIAN_POINT('Ctrl Pts',(45.160919615482,34.1797353353169,-13.6662889929718));
#11061=CARTESIAN_POINT('Ctrl Pts',(46.1678099981384,34.1587547626374,-13.4067701419416));
#11062=CARTESIAN_POINT('Ctrl Pts',(47.2697485955313,34.1358155634133,-12.99212771218));
#11063=CARTESIAN_POINT('Ctrl Pts',(47.5806825568258,34.1291168241642,-12.8439948607373));
#11064=CARTESIAN_POINT('Ctrl Pts',(47.9620635928185,34.12110612595,-12.6079631387512));
#11065=CARTESIAN_POINT('Ctrl Pts',(48.1105225594667,34.1180354578981,-12.5002738736583));
#11066=CARTESIAN_POINT('Ctrl Pts',(48.273968864556,34.1147213882706,-12.3221425525957));
#11067=CARTESIAN_POINT('Ctrl Pts',(48.3224965288387,34.1137498895631,-12.2559081706184));
#11068=CARTESIAN_POINT('Ctrl Pts',(48.3780029687333,34.1126452008863,-12.1334238063378));
#11069=CARTESIAN_POINT('Ctrl Pts',(48.3924560861139,34.112359727204,-12.0802291421916));
#11070=CARTESIAN_POINT('Ctrl Pts',(48.3995482155258,34.1122194864959,-11.9678088049197));
#11071=CARTESIAN_POINT('Ctrl Pts',(48.3907243897671,34.1123934916437,-11.9125774118326));
#11072=CARTESIAN_POINT('Ctrl Pts',(48.3454843224248,34.1132914041617,-11.7814945151571));
#11073=CARTESIAN_POINT('Ctrl Pts',(48.2991619954205,34.1142152790324,-11.7114707460069));
#11074=CARTESIAN_POINT('Ctrl Pts',(48.1374682888603,34.1174821663948,-11.5199114966352));
#11075=CARTESIAN_POINT('Ctrl Pts',(47.9801661690144,34.1207252470435,-11.4029519559693));
#11076=CARTESIAN_POINT('Ctrl Pts',(47.5679314366847,34.1293856593842,-11.1485634224112));
#11077=CARTESIAN_POINT('Ctrl Pts',(47.2511618706624,34.1362071261756,-11.0003953633426));
#11078=CARTESIAN_POINT('Ctrl Pts',(45.8398323679199,34.1655686944463,-10.4712348722153));
#11079=CARTESIAN_POINT('Ctrl Pts',(44.2829168047143,34.1970037684738,-10.1380987514247));
#11080=CARTESIAN_POINT('Ctrl Pts',(42.5,34.1970037684738,-10.1380987514247));
#11081=CARTESIAN_POINT('Origin',(50.,54.6122755947453,-11.9999999999999));
#11082=CARTESIAN_POINT('',(50.,54.6122755947453,7.50000000000009));
#11083=CARTESIAN_POINT('Origin',(50.,54.6122755947453,-11.9999999999999));
#11084=CARTESIAN_POINT('',(50.,54.6122755947453,5.50000000000008));
#11085=CARTESIAN_POINT('Origin',(50.,54.6122755947453,-11.9999999999999));
#11086=CARTESIAN_POINT('Origin',(35.,54.6122755947453,-11.9999999999999));
#11087=CARTESIAN_POINT('',(35.,54.6122755947453,7.50000000000008));
#11088=CARTESIAN_POINT('Origin',(35.,54.6122755947453,-11.9999999999999));
#11089=CARTESIAN_POINT('',(35.,54.6122755947453,5.50000000000008));
#11090=CARTESIAN_POINT('Origin',(35.,54.6122755947453,-11.9999999999999));
#11091=CARTESIAN_POINT('Ctrl Pts',(36.6000954047721,75.6303323723191,-11.0710623055408));
#11092=CARTESIAN_POINT('Ctrl Pts',(36.6000954047721,75.1163129851934,-11.390036451076));
#11093=CARTESIAN_POINT('Ctrl Pts',(36.6000954047721,75.113533389205,-11.9949767040821));
#11094=CARTESIAN_POINT('Ctrl Pts',(36.6000954047721,75.1107537932165,-12.5999169570882));
#11095=CARTESIAN_POINT('Ctrl Pts',(36.6000954047721,75.6218202760576,-12.923601195162));
#11096=CARTESIAN_POINT('Ctrl Pts',(42.4997945641984,74.4160919611753,-9.11434223685902));
#11097=CARTESIAN_POINT('Ctrl Pts',(42.4997945641984,72.8193389779435,-10.1052054829035));
#11098=CARTESIAN_POINT('Ctrl Pts',(42.4997945641984,72.8107044238821,-11.9843956026886));
#11099=CARTESIAN_POINT('Ctrl Pts',(42.4997945641984,72.8020698698207,-13.8635857224736));
#11100=CARTESIAN_POINT('Ctrl Pts',(42.4997945641984,74.3896499330349,-14.8690804289273));
#11101=CARTESIAN_POINT('Ctrl Pts',(48.3995480441881,75.630258991695,-11.0709440543786));
#11102=CARTESIAN_POINT('Ctrl Pts',(48.3995480441881,75.1161741713435,-11.3899588044276));
#11103=CARTESIAN_POINT('Ctrl Pts',(48.3995480441881,75.1133942215203,-11.9949760646306));
#11104=CARTESIAN_POINT('Ctrl Pts',(48.3995480441881,75.1106142716971,-12.5999933248336));
#11105=CARTESIAN_POINT('Ctrl Pts',(48.3995480441881,75.6217458118676,-12.9237187670028));
#11106=CARTESIAN_POINT('Ctrl Pts',(36.6000954047721,53.6833379002862,9.01805677757378));
#11107=CARTESIAN_POINT('Ctrl Pts',(36.6000954047721,54.0023120458214,8.50403739044816));
#11108=CARTESIAN_POINT('Ctrl Pts',(36.6000954047721,54.6072522988275,8.50125779445973));
#11109=CARTESIAN_POINT('Ctrl Pts',(36.6000954047721,55.2121925518336,8.4984781984713));
#11110=CARTESIAN_POINT('Ctrl Pts',(36.6000954047721,55.5358767899073,9.00954468131236));
#11111=CARTESIAN_POINT('Ctrl Pts',(42.4997945641984,51.7266178316045,7.80381636642986));
#11112=CARTESIAN_POINT('Ctrl Pts',(42.4997945641984,52.7174810776491,6.2070633831982));
#11113=CARTESIAN_POINT('Ctrl Pts',(42.4997945641984,54.596671197434,6.19842882913689));
#11114=CARTESIAN_POINT('Ctrl Pts',(42.4997945641984,56.4758613172189,6.18979427507558));
#11115=CARTESIAN_POINT('Ctrl Pts',(42.4997945641984,57.4813560236726,7.77737433828968));
#11116=CARTESIAN_POINT('Ctrl Pts',(48.3995480441881,53.683219649124,9.0179833969497));
#11117=CARTESIAN_POINT('Ctrl Pts',(48.3995480441881,54.002234399173,8.50389857659829));
#11118=CARTESIAN_POINT('Ctrl Pts',(48.3995480441881,54.607251659376,8.50111862677509));
#11119=CARTESIAN_POINT('Ctrl Pts',(48.3995480441881,55.212268919579,8.49833867695189));
#11120=CARTESIAN_POINT('Ctrl Pts',(48.3995480441881,55.5359943617481,9.00947021712231));
#11121=CARTESIAN_POINT('Ctrl Pts',(36.6000954047722,33.5942188171715,-12.9289376944591));
#11122=CARTESIAN_POINT('Ctrl Pts',(36.6000954047722,34.1082382042972,-12.6099635489239));
#11123=CARTESIAN_POINT('Ctrl Pts',(36.6000954047722,34.1110178002857,-12.0050232959178));
#11124=CARTESIAN_POINT('Ctrl Pts',(36.6000954047722,34.1137973962741,-11.4000830429116));
#11125=CARTESIAN_POINT('Ctrl Pts',(36.6000954047722,33.602730913433,-11.0763988048379));
#11126=CARTESIAN_POINT('Ctrl Pts',(42.4997945641985,34.8084592283153,-14.8856577631409));
#11127=CARTESIAN_POINT('Ctrl Pts',(42.4997945641985,36.4052122115471,-13.8947945170964));
#11128=CARTESIAN_POINT('Ctrl Pts',(42.4997945641985,36.4138467656085,-12.0156043973113));
#11129=CARTESIAN_POINT('Ctrl Pts',(42.4997945641985,36.4224813196699,-10.1364142775263));
#11130=CARTESIAN_POINT('Ctrl Pts',(42.4997945641985,34.8349012564557,-9.13091957107256));
#11131=CARTESIAN_POINT('Ctrl Pts',(48.3995480441881,33.5942921977956,-12.9290559456212));
#11132=CARTESIAN_POINT('Ctrl Pts',(48.3995480441881,34.1083770181471,-12.6100411955723));
#11133=CARTESIAN_POINT('Ctrl Pts',(48.3995480441881,34.1111569679703,-12.0050239353692));
#11134=CARTESIAN_POINT('Ctrl Pts',(48.3995480441881,34.1139369177935,-11.4000066751662));
#11135=CARTESIAN_POINT('Ctrl Pts',(48.3995480441881,33.6028053776231,-11.0762812329971));
#11136=CARTESIAN_POINT('Ctrl Pts',(36.603289189263,55.5369296408085,-33.0088778576148));
#11137=CARTESIAN_POINT('Ctrl Pts',(36.603289189263,55.2128764217899,-32.4972287891192));
#11138=CARTESIAN_POINT('Ctrl Pts',(36.603289189263,54.6072465725666,-32.5000115536831));
#11139=CARTESIAN_POINT('Ctrl Pts',(36.603289189263,54.0016167233433,-32.5027943182471));
#11140=CARTESIAN_POINT('Ctrl Pts',(36.603289189263,53.682278966091,-33.0173996571641));
#11141=CARTESIAN_POINT('Ctrl Pts',(42.5,57.4802106040728,-31.7780997904234));
#11142=CARTESIAN_POINT('Ctrl Pts',(42.5,56.4751173200863,-30.1911535349279));
#11143=CARTESIAN_POINT('Ctrl Pts',(42.5,54.5966774271594,-30.1997846418264));
#11144=CARTESIAN_POINT('Ctrl Pts',(42.5,52.7182375342324,-30.2084157487249));
#11145=CARTESIAN_POINT('Ctrl Pts',(42.5,51.7277698693544,-31.8045312621439));
#11146=CARTESIAN_POINT('Ctrl Pts',(48.396710810737,55.5369296408085,-33.0088778576148));
#11147=CARTESIAN_POINT('Ctrl Pts',(48.396710810737,55.2128764217899,-32.4972287891192));
#11148=CARTESIAN_POINT('Ctrl Pts',(48.396710810737,54.6072465725666,-32.5000115536831));
#11149=CARTESIAN_POINT('Ctrl Pts',(48.396710810737,54.0016167233433,-32.5027943182471));
#11150=CARTESIAN_POINT('Ctrl Pts',(48.396710810737,53.682278966091,-33.0173996571641));
#11151=CARTESIAN_POINT('Origin',(47.5,69.4571012113211,2.84482561657582));
#11152=CARTESIAN_POINT('',(47.5,70.4387355541152,2.55242815321436));
#11153=CARTESIAN_POINT('',(47.5,69.1647037479597,3.82645995936986));
#11154=CARTESIAN_POINT('Origin',(47.5,69.4571012113211,2.84482561657582));
#11155=CARTESIAN_POINT('',(47.537899429919,70.3143910047143,2.28432898886365));
#11156=CARTESIAN_POINT('Ctrl Pts',(47.5,70.4387355541152,2.55242815321436));
#11157=CARTESIAN_POINT('Ctrl Pts',(47.5,70.4189527998948,2.48601365455714));
#11158=CARTESIAN_POINT('Ctrl Pts',(47.5053044417601,70.3925771182096,2.422112506851));
#11159=CARTESIAN_POINT('Ctrl Pts',(47.5230476022983,70.3458637388305,2.33479395638985));
#11160=CARTESIAN_POINT('Ctrl Pts',(47.5298073931343,70.3305302530218,2.30901426289197));
#11161=CARTESIAN_POINT('Ctrl Pts',(47.537899429919,70.3143910047143,2.28432898886365));
#11162=CARTESIAN_POINT('',(37.4621005700809,70.3143910047143,2.28432898886365));
#11163=CARTESIAN_POINT('',(47.537899429919,70.3143910047143,2.28432898886365));
#11164=CARTESIAN_POINT('',(37.5,70.4387355541152,2.55242815321436));
#11165=CARTESIAN_POINT('Ctrl Pts',(37.462100570081,70.3143910047143,2.28432898886366));
#11166=CARTESIAN_POINT('Ctrl Pts',(37.4632744099609,70.3167321820717,2.28790986224227));
#11167=CARTESIAN_POINT('Ctrl Pts',(37.4644207388779,70.3190574281895,2.29151535342116));
#11168=CARTESIAN_POINT('Ctrl Pts',(37.4898409184866,70.371513910436,2.37399296978792));
#11169=CARTESIAN_POINT('Ctrl Pts',(37.5,70.4113518729136,2.46049588543571));
#11170=CARTESIAN_POINT('Ctrl Pts',(37.5,70.4387355541152,2.55242815321435));
#11171=CARTESIAN_POINT('',(37.5,69.1647037479597,3.82645995936986));
#11172=CARTESIAN_POINT('Origin',(37.5,69.4571012113211,2.84482561657581));
#11173=CARTESIAN_POINT('',(37.4621005700809,68.8966045836089,3.70211540996904));
#11174=CARTESIAN_POINT('Ctrl Pts',(37.5,69.1647037479597,3.82645995936986));
#11175=CARTESIAN_POINT('Ctrl Pts',(37.5,69.0990912208333,3.80691608680946));
#11176=CARTESIAN_POINT('Ctrl Pts',(37.4948229521317,69.0359160073849,3.78093293985881));
#11177=CARTESIAN_POINT('Ctrl Pts',(37.4773121076774,68.948446705185,3.73440602894735));
#11178=CARTESIAN_POINT('Ctrl Pts',(37.470409170669,68.9219504993238,3.7186865862433));
#11179=CARTESIAN_POINT('Ctrl Pts',(37.462100570081,68.896604583609,3.70211540996904));
#11180=CARTESIAN_POINT('',(47.5378994299191,68.8966045836089,3.70211540996904));
#11181=CARTESIAN_POINT('',(47.5378994299191,68.8966045836089,3.70211540996904));
#11182=CARTESIAN_POINT('Ctrl Pts',(47.537899429919,68.8966045836089,3.70211540996903));
#11183=CARTESIAN_POINT('Ctrl Pts',(47.5369318666484,68.8995561970421,3.7040451767624));
#11184=CARTESIAN_POINT('Ctrl Pts',(47.5359829808858,68.9025245795757,3.7059641473824));
#11185=CARTESIAN_POINT('Ctrl Pts',(47.510332174293,68.9848409778267,3.75857431922063));
#11186=CARTESIAN_POINT('Ctrl Pts',(47.5,69.0719944289914,3.79884481948067));
#11187=CARTESIAN_POINT('Ctrl Pts',(47.5,69.1647037479597,3.82645995936986));
#11188=CARTESIAN_POINT('Origin',(47.5,54.6122755947453,-11.9999999999999));
#11189=CARTESIAN_POINT('Origin',(47.5,54.6122755947453,-11.9999999999999));
#11190=CARTESIAN_POINT('Origin',(37.5,54.6122755947453,-11.9999999999999));
#11191=CARTESIAN_POINT('Origin',(37.5,54.6122755947453,-11.9999999999999));
#11192=CARTESIAN_POINT('Origin',(47.5,68.349381898499,4.5391024665601));
#11193=CARTESIAN_POINT('Ctrl Pts',(37.4621005700809,68.896604583609,3.70211540996902));
#11194=CARTESIAN_POINT('Ctrl Pts',(37.4310083838403,68.8017558875511,3.6401032704416));
#11195=CARTESIAN_POINT('Ctrl Pts',(37.3828779782886,68.7018867262922,3.59772631179564));
#11196=CARTESIAN_POINT('Ctrl Pts',(37.245031822289,68.4694900791145,3.53679150015867));
#11197=CARTESIAN_POINT('Ctrl Pts',(37.1423703640038,68.3305669520952,3.52988534954539));
#11198=CARTESIAN_POINT('Ctrl Pts',(36.8667626334574,68.017493954875,3.57885731564907));
#11199=CARTESIAN_POINT('Ctrl Pts',(36.6872103879512,67.8515747651484,3.65364745765698));
#11200=CARTESIAN_POINT('Ctrl Pts',(36.5029780432796,67.7126857281249,3.76798632698662));
#11201=CARTESIAN_POINT('Ctrl Pts',(36.5014890205786,67.711565210995,3.76891288782061));
#11202=CARTESIAN_POINT('Ctrl Pts',(36.5,67.7104467215802,3.76984188672011));
#11203=CARTESIAN_POINT('Ctrl Pts',(47.537899429919,68.896604583609,3.70211540996901));
#11204=CARTESIAN_POINT('Ctrl Pts',(47.5689916161593,68.8017558875522,3.64010327044235));
#11205=CARTESIAN_POINT('Ctrl Pts',(47.6171220217102,68.7018867262946,3.59772631179665));
#11206=CARTESIAN_POINT('Ctrl Pts',(47.7549681777082,68.4694900791187,3.53679150015924));
#11207=CARTESIAN_POINT('Ctrl Pts',(47.8576296359926,68.3305669520998,3.52988534954533));
#11208=CARTESIAN_POINT('Ctrl Pts',(48.1332373665856,68.0174939548254,3.57885731565596));
#11209=CARTESIAN_POINT('Ctrl Pts',(48.3127896121225,67.8515747651177,3.65364745768193));
#11210=CARTESIAN_POINT('Ctrl Pts',(48.4970219567203,67.7126857281242,3.76798632698724));
#11211=CARTESIAN_POINT('Ctrl Pts',(48.498510979422,67.7115652109945,3.76891288782097));
#11212=CARTESIAN_POINT('Ctrl Pts',(48.5,67.7104467215802,3.7698418867201));
#11213=CARTESIAN_POINT('Origin',(48.5,54.6122755947453,-11.9999999999999));
#11214=CARTESIAN_POINT('Ctrl Pts',(47.537899429919,70.3143910047143,2.28432898886365));
#11215=CARTESIAN_POINT('Ctrl Pts',(47.5689916161588,70.2523788651886,2.18948029280836));
#11216=CARTESIAN_POINT('Ctrl Pts',(47.6171220217088,70.2100019065432,2.08961113155225));
#11217=CARTESIAN_POINT('Ctrl Pts',(47.7549681777051,70.1490670949051,1.85721448437786));
#11218=CARTESIAN_POINT('Ctrl Pts',(47.8576296359887,70.1421609442907,1.71829135735951));
#11219=CARTESIAN_POINT('Ctrl Pts',(48.1332373666213,70.1911329104067,1.40521836003877));
#11220=CARTESIAN_POINT('Ctrl Pts',(48.3127896121854,70.2659230524474,1.23929917034817));
#11221=CARTESIAN_POINT('Ctrl Pts',(48.4970219567186,70.3802619217321,1.10041013337938));
#11222=CARTESIAN_POINT('Ctrl Pts',(48.4985109794219,70.3811884825662,1.09928961624927));
#11223=CARTESIAN_POINT('Ctrl Pts',(48.5,70.3821174814654,1.09817112683487));
#11224=CARTESIAN_POINT('Origin',(36.5,54.6122755947453,-11.9999999999999));
#11225=CARTESIAN_POINT('Ctrl Pts',(37.4621005700809,70.3143910047143,2.28432898886365));
#11226=CARTESIAN_POINT('Ctrl Pts',(37.4310083838412,70.2523788651887,2.18948029280845));
#11227=CARTESIAN_POINT('Ctrl Pts',(37.3828779782913,70.2100019065433,2.08961113155242));
#11228=CARTESIAN_POINT('Ctrl Pts',(37.2450318222954,70.1490670949052,1.85721448437858));
#11229=CARTESIAN_POINT('Ctrl Pts',(37.1423703640119,70.1421609442906,1.71829135736027));
#11230=CARTESIAN_POINT('Ctrl Pts',(36.8667626333773,70.1911329104068,1.40521836003708));
#11231=CARTESIAN_POINT('Ctrl Pts',(36.6872103878129,70.2659230524489,1.23929917034637));
#11232=CARTESIAN_POINT('Ctrl Pts',(36.5029780432807,70.3802619217326,1.10041013337885));
#11233=CARTESIAN_POINT('Ctrl Pts',(36.5014890205792,70.3811884825656,1.09928961625003));
#11234=CARTESIAN_POINT('Ctrl Pts',(36.5,70.3821174814654,1.09817112683487));
#11235=CARTESIAN_POINT('Origin',(50.,71.1513780613054,1.73710630375365));
#11236=CARTESIAN_POINT('Origin',(47.5,39.7674499781698,2.84482561657604));
#11237=CARTESIAN_POINT('',(47.5,40.0598474415312,3.82645995937007));
#11238=CARTESIAN_POINT('',(47.5,38.7858156353757,2.5524281532146));
#11239=CARTESIAN_POINT('Origin',(47.5,39.7674499781698,2.84482561657604));
#11240=CARTESIAN_POINT('',(47.5378994299191,40.3279466058819,3.70211540996925));
#11241=CARTESIAN_POINT('Ctrl Pts',(47.5,40.0598474415312,3.82645995937007));
#11242=CARTESIAN_POINT('Ctrl Pts',(47.5,40.1262619401886,3.80667720514962));
#11243=CARTESIAN_POINT('Ctrl Pts',(47.5053044417602,40.1901630878949,3.7803015234644));
#11244=CARTESIAN_POINT('Ctrl Pts',(47.5230476022984,40.277481638356,3.73358814408523));
#11245=CARTESIAN_POINT('Ctrl Pts',(47.5298073931343,40.3032613318537,3.71825465827663));
#11246=CARTESIAN_POINT('Ctrl Pts',(47.537899429919,40.3279466058819,3.70211540996925));
#11247=CARTESIAN_POINT('',(37.462100570081,40.3279466058819,3.70211540996925));
#11248=CARTESIAN_POINT('',(47.5378994299191,40.3279466058819,3.70211540996925));
#11249=CARTESIAN_POINT('',(37.5,40.0598474415312,3.82645995937007));
#11250=CARTESIAN_POINT('Ctrl Pts',(37.462100570081,40.3279466058819,3.70211540996925));
#11251=CARTESIAN_POINT('Ctrl Pts',(37.4632744099609,40.3243657325033,3.70445658732663));
#11252=CARTESIAN_POINT('Ctrl Pts',(37.4644207388779,40.3207602413243,3.70678183344449));
#11253=CARTESIAN_POINT('Ctrl Pts',(37.4898409184866,40.2382826249574,3.75923831569102));
#11254=CARTESIAN_POINT('Ctrl Pts',(37.5,40.1517797093097,3.7990762781686));
#11255=CARTESIAN_POINT('Ctrl Pts',(37.5,40.0598474415312,3.82645995937007));
#11256=CARTESIAN_POINT('',(37.5,38.7858156353757,2.55242815321459));
#11257=CARTESIAN_POINT('Origin',(37.5,39.7674499781698,2.84482561657603));
#11258=CARTESIAN_POINT('',(37.462100570081,38.9101601847765,2.28432898886388));
#11259=CARTESIAN_POINT('Ctrl Pts',(37.5,38.7858156353757,2.55242815321459));
#11260=CARTESIAN_POINT('Ctrl Pts',(37.5,38.8053595079361,2.48681562608814));
#11261=CARTESIAN_POINT('Ctrl Pts',(37.4948229521316,38.8313426548868,2.42364041263967));
#11262=CARTESIAN_POINT('Ctrl Pts',(37.4773121076774,38.8778695657982,2.33617111043986));
#11263=CARTESIAN_POINT('Ctrl Pts',(37.470409170669,38.8935890085023,2.3096749045787));
#11264=CARTESIAN_POINT('Ctrl Pts',(37.462100570081,38.9101601847765,2.28432898886388));
#11265=CARTESIAN_POINT('',(47.5378994299191,38.9101601847765,2.28432898886388));
#11266=CARTESIAN_POINT('',(47.5378994299191,38.9101601847765,2.28432898886388));
#11267=CARTESIAN_POINT('Ctrl Pts',(47.537899429919,38.9101601847765,2.28432898886389));
#11268=CARTESIAN_POINT('Ctrl Pts',(47.5369318666484,38.9082304179831,2.28728060229702));
#11269=CARTESIAN_POINT('Ctrl Pts',(47.5359829808858,38.9063114473632,2.29024898483066));
#11270=CARTESIAN_POINT('Ctrl Pts',(47.5103321742929,38.8537012755249,2.37256538308168));
#11271=CARTESIAN_POINT('Ctrl Pts',(47.5,38.8134307752649,2.45971883424642));
#11272=CARTESIAN_POINT('Ctrl Pts',(47.5,38.7858156353757,2.5524281532146));
#11273=CARTESIAN_POINT('Origin',(47.5,54.6122755947453,-11.9999999999999));
#11274=CARTESIAN_POINT('Origin',(47.5,54.6122755947453,-11.9999999999999));
#11275=CARTESIAN_POINT('Origin',(37.5,54.6122755947453,-11.9999999999999));
#11276=CARTESIAN_POINT('Origin',(37.5,54.6122755947453,-11.9999999999999));
#11277=CARTESIAN_POINT('Origin',(47.5,39.7674499781695,-26.8448256165756));
#11278=CARTESIAN_POINT('',(47.5,38.7858156353755,-26.5524281532142));
#11279=CARTESIAN_POINT('',(47.5,40.059847441531,-27.8264599593697));
#11280=CARTESIAN_POINT('Origin',(47.5,39.7674499781695,-26.8448256165756));
#11281=CARTESIAN_POINT('',(47.5378994299191,38.9101601847763,-26.2843289888635));
#11282=CARTESIAN_POINT('Ctrl Pts',(47.5,38.7858156353755,-26.5524281532142));
#11283=CARTESIAN_POINT('Ctrl Pts',(47.5,38.8055983895958,-26.4860136545571));
#11284=CARTESIAN_POINT('Ctrl Pts',(47.5053044417601,38.8319740712809,-26.4221125068513));
#11285=CARTESIAN_POINT('Ctrl Pts',(47.5230476022982,38.8786874506599,-26.3347939563902));
#11286=CARTESIAN_POINT('Ctrl Pts',(47.5298073931342,38.8940209364687,-26.309014262892));
#11287=CARTESIAN_POINT('Ctrl Pts',(47.5378994299191,38.9101601847763,-26.2843289888635));
#11288=CARTESIAN_POINT('',(37.462100570081,38.9101601847763,-26.2843289888635));
#11289=CARTESIAN_POINT('',(47.5378994299191,38.9101601847763,-26.2843289888635));
#11290=CARTESIAN_POINT('',(37.5,38.7858156353755,-26.5524281532142));
#11291=CARTESIAN_POINT('Ctrl Pts',(37.462100570081,38.9101601847763,-26.2843289888635));
#11292=CARTESIAN_POINT('Ctrl Pts',(37.463274409961,38.9078190074188,-26.2879098622423));
#11293=CARTESIAN_POINT('Ctrl Pts',(37.464420738878,38.9054937613009,-26.2915153534214));
#11294=CARTESIAN_POINT('Ctrl Pts',(37.4898409184867,38.8530372790542,-26.3739929697886));
#11295=CARTESIAN_POINT('Ctrl Pts',(37.5,38.8131993165768,-26.4604958854362));
#11296=CARTESIAN_POINT('Ctrl Pts',(37.5,38.7858156353755,-26.5524281532142));
#11297=CARTESIAN_POINT('',(37.5,40.059847441531,-27.8264599593697));
#11298=CARTESIAN_POINT('Origin',(37.5,39.7674499781695,-26.8448256165756));
#11299=CARTESIAN_POINT('',(37.462100570081,40.3279466058817,-27.7021154099689));
#11300=CARTESIAN_POINT('Ctrl Pts',(37.5,40.059847441531,-27.8264599593697));
#11301=CARTESIAN_POINT('Ctrl Pts',(37.5,40.1254599686575,-27.8069160868092));
#11302=CARTESIAN_POINT('Ctrl Pts',(37.4948229521316,40.1886351821059,-27.7809329398586));
#11303=CARTESIAN_POINT('Ctrl Pts',(37.4773121076774,40.2761044843057,-27.7344060289472));
#11304=CARTESIAN_POINT('Ctrl Pts',(37.470409170669,40.3026006901669,-27.7186865862431));
#11305=CARTESIAN_POINT('Ctrl Pts',(37.462100570081,40.3279466058817,-27.7021154099689));
#11306=CARTESIAN_POINT('',(47.5378994299191,40.3279466058817,-27.7021154099689));
#11307=CARTESIAN_POINT('',(47.5378994299191,40.3279466058817,-27.7021154099689));
#11308=CARTESIAN_POINT('Ctrl Pts',(47.5378994299191,40.3279466058817,-27.7021154099689));
#11309=CARTESIAN_POINT('Ctrl Pts',(47.5369318666484,40.3249949924486,-27.7040451767622));
#11310=CARTESIAN_POINT('Ctrl Pts',(47.5359829808858,40.3220266099149,-27.7059641473822));
#11311=CARTESIAN_POINT('Ctrl Pts',(47.5103321742929,40.2397102116637,-27.7585743192207));
#11312=CARTESIAN_POINT('Ctrl Pts',(47.5,40.1525567604989,-27.7988448194806));
#11313=CARTESIAN_POINT('Ctrl Pts',(47.5,40.059847441531,-27.8264599593697));
#11314=CARTESIAN_POINT('Origin',(47.5,54.6122755947453,-11.9999999999999));
#11315=CARTESIAN_POINT('Origin',(47.5,54.6122755947453,-11.9999999999999));
#11316=CARTESIAN_POINT('Origin',(37.5,54.6122755947453,-11.9999999999999));
#11317=CARTESIAN_POINT('Origin',(37.5,54.6122755947453,-11.9999999999999));
#11318=CARTESIAN_POINT('Origin',(47.5,69.457101211321,-26.8448256165758));
#11319=CARTESIAN_POINT('',(47.5,69.1647037479595,-27.8264599593698));
#11320=CARTESIAN_POINT('',(47.5,70.4387355541151,-26.5524281532143));
#11321=CARTESIAN_POINT('Origin',(47.5,69.457101211321,-26.8448256165758));
#11322=CARTESIAN_POINT('',(47.5378994299191,68.8966045836088,-27.702115409969));
#11323=CARTESIAN_POINT('Ctrl Pts',(47.5,69.1647037479595,-27.8264599593698));
#11324=CARTESIAN_POINT('Ctrl Pts',(47.5,69.0982892493024,-27.8066772051495));
#11325=CARTESIAN_POINT('Ctrl Pts',(47.5053044417601,69.0343881015963,-27.7803015234644));
#11326=CARTESIAN_POINT('Ctrl Pts',(47.5230476022983,68.9470695511352,-27.7335881440852));
#11327=CARTESIAN_POINT('Ctrl Pts',(47.5298073931342,68.9212898576372,-27.7182546582765));
#11328=CARTESIAN_POINT('Ctrl Pts',(47.5378994299191,68.8966045836088,-27.702115409969));
#11329=CARTESIAN_POINT('',(37.462100570081,68.8966045836088,-27.702115409969));
#11330=CARTESIAN_POINT('',(47.5378994299191,68.8966045836088,-27.702115409969));
#11331=CARTESIAN_POINT('',(37.5,69.1647037479595,-27.8264599593698));
#11332=CARTESIAN_POINT('Ctrl Pts',(37.462100570081,68.8966045836088,-27.702115409969));
#11333=CARTESIAN_POINT('Ctrl Pts',(37.4632744099607,68.900185456987,-27.704456587326));
#11334=CARTESIAN_POINT('Ctrl Pts',(37.4644207388776,68.9037909481654,-27.7067818334436));
#11335=CARTESIAN_POINT('Ctrl Pts',(37.4898409184865,68.9862685645324,-27.7592383156903));
#11336=CARTESIAN_POINT('Ctrl Pts',(37.5,69.0727714801806,-27.7990762781682));
#11337=CARTESIAN_POINT('Ctrl Pts',(37.5,69.1647037479595,-27.8264599593698));
#11338=CARTESIAN_POINT('',(37.5,70.4387355541151,-26.5524281532143));
#11339=CARTESIAN_POINT('Origin',(37.5,69.457101211321,-26.8448256165758));
#11340=CARTESIAN_POINT('',(37.462100570081,70.3143910047142,-26.2843289888636));
#11341=CARTESIAN_POINT('Ctrl Pts',(37.5,70.4387355541151,-26.5524281532143));
#11342=CARTESIAN_POINT('Ctrl Pts',(37.5,70.4191916815546,-26.4868156260878));
#11343=CARTESIAN_POINT('Ctrl Pts',(37.4948229521316,70.3932085346039,-26.4236404126394));
#11344=CARTESIAN_POINT('Ctrl Pts',(37.4773121076774,70.3466816236925,-26.3361711104396));
#11345=CARTESIAN_POINT('Ctrl Pts',(37.470409170669,70.3309621809885,-26.3096749045784));
#11346=CARTESIAN_POINT('Ctrl Pts',(37.462100570081,70.3143910047142,-26.2843289888636));
#11347=CARTESIAN_POINT('',(47.5378994299191,70.3143910047142,-26.2843289888636));
#11348=CARTESIAN_POINT('',(47.5378994299191,70.3143910047142,-26.2843289888636));
#11349=CARTESIAN_POINT('Ctrl Pts',(47.5378994299191,70.3143910047142,-26.2843289888636));
#11350=CARTESIAN_POINT('Ctrl Pts',(47.5369318666484,70.3163207715076,-26.2872806022967));
#11351=CARTESIAN_POINT('Ctrl Pts',(47.5359829808858,70.3182397421275,-26.2902489848303));
#11352=CARTESIAN_POINT('Ctrl Pts',(47.510332174293,70.3708499139657,-26.3725653830812));
#11353=CARTESIAN_POINT('Ctrl Pts',(47.5,70.4111204142258,-26.4597188342459));
#11354=CARTESIAN_POINT('Ctrl Pts',(47.5,70.4387355541151,-26.5524281532143));
#11355=CARTESIAN_POINT('Origin',(47.5,54.6122755947453,-11.9999999999999));
#11356=CARTESIAN_POINT('Origin',(47.5,54.6122755947453,-11.9999999999999));
#11357=CARTESIAN_POINT('Origin',(37.5,54.6122755947453,-11.9999999999999));
#11358=CARTESIAN_POINT('Origin',(37.5,54.6122755947453,-11.9999999999999));
#11359=CARTESIAN_POINT('Origin',(47.5,71.1513780613053,-25.7371063037536));
#11360=CARTESIAN_POINT('Ctrl Pts',(37.462100570081,70.3143910047142,-26.2843289888636));
#11361=CARTESIAN_POINT('Ctrl Pts',(37.4310083838417,70.2523788651895,-26.1894802928099));
#11362=CARTESIAN_POINT('Ctrl Pts',(37.3828779782928,70.2100019065445,-26.0896111315555));
#11363=CARTESIAN_POINT('Ctrl Pts',(37.2450318222992,70.1490670949059,-25.8572144843843));
#11364=CARTESIAN_POINT('Ctrl Pts',(37.1423703640169,70.1421609442904,-25.7182913573665));
#11365=CARTESIAN_POINT('Ctrl Pts',(36.8667626333183,70.1911329104162,-25.4052183599692));
#11366=CARTESIAN_POINT('Ctrl Pts',(36.6872103877121,70.2659230524829,-25.2392991703043));
#11367=CARTESIAN_POINT('Ctrl Pts',(36.5029780432812,70.3802619217331,-25.1004101333781));
#11368=CARTESIAN_POINT('Ctrl Pts',(36.5014890205775,70.3811884825665,-25.0992896162488));
#11369=CARTESIAN_POINT('Ctrl Pts',(36.5,70.3821174814653,-25.0981711268349));
#11370=CARTESIAN_POINT('Ctrl Pts',(47.5378994299191,70.3143910047142,-26.2843289888636));
#11371=CARTESIAN_POINT('Ctrl Pts',(47.568991616158,70.2523788651901,-26.1894802928108));
#11372=CARTESIAN_POINT('Ctrl Pts',(47.6171220217063,70.2100019065453,-26.0896111315574));
#11373=CARTESIAN_POINT('Ctrl Pts',(47.7549681776988,70.1490670949063,-25.8572144843871));
#11374=CARTESIAN_POINT('Ctrl Pts',(47.8576296359807,70.1421609442904,-25.7182913573697));
#11375=CARTESIAN_POINT('Ctrl Pts',(48.1332373667109,70.1911329104208,-25.4052183599355));
#11376=CARTESIAN_POINT('Ctrl Pts',(48.3127896123394,70.2659230524989,-25.2392991702846));
#11377=CARTESIAN_POINT('Ctrl Pts',(48.4970219567185,70.3802619217334,-25.1004101333777));
#11378=CARTESIAN_POINT('Ctrl Pts',(48.4985109794227,70.3811884825666,-25.0992896162486));
#11379=CARTESIAN_POINT('Ctrl Pts',(48.5,70.3821174814653,-25.0981711268349));
#11380=CARTESIAN_POINT('Origin',(48.5,54.6122755947453,-11.9999999999999));
#11381=CARTESIAN_POINT('Ctrl Pts',(47.5378994299191,68.8966045836088,-27.702115409969));
#11382=CARTESIAN_POINT('Ctrl Pts',(47.5689916161593,68.8017558875521,-27.6401032704423));
#11383=CARTESIAN_POINT('Ctrl Pts',(47.6171220217102,68.7018867262945,-27.5977263117966));
#11384=CARTESIAN_POINT('Ctrl Pts',(47.7549681777078,68.4694900791192,-27.5367915001594));
#11385=CARTESIAN_POINT('Ctrl Pts',(47.857629635992,68.3305669521004,-27.5298853495452));
#11386=CARTESIAN_POINT('Ctrl Pts',(48.1332373665661,68.0174939548474,-27.5788573156524));
#11387=CARTESIAN_POINT('Ctrl Pts',(48.3127896120915,67.8515747651331,-27.6536474576698));
#11388=CARTESIAN_POINT('Ctrl Pts',(48.4970219567174,67.7126857281265,-27.7679863269852));
#11389=CARTESIAN_POINT('Ctrl Pts',(48.4985109794222,67.7115652109942,-27.7689128878211));
#11390=CARTESIAN_POINT('Ctrl Pts',(48.5,67.71044672158,-27.7698418867201));
#11391=CARTESIAN_POINT('Origin',(36.5,54.6122755947453,-11.9999999999999));
#11392=CARTESIAN_POINT('Ctrl Pts',(37.462100570081,68.8966045836088,-27.702115409969));
#11393=CARTESIAN_POINT('Ctrl Pts',(37.4310083838413,68.8017558875538,-27.6401032704434));
#11394=CARTESIAN_POINT('Ctrl Pts',(37.3828779782915,68.701886726298,-27.5977263117981));
#11395=CARTESIAN_POINT('Ctrl Pts',(37.245031822296,68.4694900791247,-27.5367915001601));
#11396=CARTESIAN_POINT('Ctrl Pts',(37.1423703640128,68.3305669521065,-27.5298853495452));
#11397=CARTESIAN_POINT('Ctrl Pts',(36.8667626333661,68.0174939547694,-27.5788573156634));
#11398=CARTESIAN_POINT('Ctrl Pts',(36.6872103877933,67.8515747650841,-27.6536474577095));
#11399=CARTESIAN_POINT('Ctrl Pts',(36.5029780432822,67.7126857281249,-27.7679863269865));
#11400=CARTESIAN_POINT('Ctrl Pts',(36.5014890205769,67.7115652109935,-27.7689128878217));
#11401=CARTESIAN_POINT('Ctrl Pts',(36.5,67.71044672158,-27.7698418867201));
#11402=CARTESIAN_POINT('Origin',(50.,68.3493818984988,-28.5391024665601));
#11403=CARTESIAN_POINT('Origin',(47.5,40.8751692909917,-28.5391024665599));
#11404=CARTESIAN_POINT('Ctrl Pts',(37.462100570081,40.3279466058817,-27.7021154099689));
#11405=CARTESIAN_POINT('Ctrl Pts',(37.4310083838416,40.4227953019356,-27.640103270444));
#11406=CARTESIAN_POINT('Ctrl Pts',(37.3828779782926,40.5226644631903,-27.5977263117989));
#11407=CARTESIAN_POINT('Ctrl Pts',(37.2450318222986,40.755061110362,-27.5367915001605));
#11408=CARTESIAN_POINT('Ctrl Pts',(37.1423703640161,40.8939842373798,-27.529885349545));
#11409=CARTESIAN_POINT('Ctrl Pts',(36.8667626333263,41.2070572347668,-27.5788573156696));
#11410=CARTESIAN_POINT('Ctrl Pts',(36.6872103877253,41.3729764244348,-27.6536474577325));
#11411=CARTESIAN_POINT('Ctrl Pts',(36.5029780432813,41.511865461367,-27.7679863269875));
#11412=CARTESIAN_POINT('Ctrl Pts',(36.5014890205774,41.5129859784966,-27.7689128878212));
#11413=CARTESIAN_POINT('Ctrl Pts',(36.5,41.5141044679104,-27.7698418867199));
#11414=CARTESIAN_POINT('Ctrl Pts',(47.5378994299191,40.3279466058817,-27.7021154099689));
#11415=CARTESIAN_POINT('Ctrl Pts',(47.5689916161584,40.4227953019356,-27.640103270444));
#11416=CARTESIAN_POINT('Ctrl Pts',(47.6171220217074,40.5226644631902,-27.597726311799));
#11417=CARTESIAN_POINT('Ctrl Pts',(47.7549681777013,40.7550611103619,-27.5367915001605));
#11418=CARTESIAN_POINT('Ctrl Pts',(47.8576296359839,40.8939842373797,-27.5298853495451));
#11419=CARTESIAN_POINT('Ctrl Pts',(48.1332373666762,41.2070572347697,-27.57885731567));
#11420=CARTESIAN_POINT('Ctrl Pts',(48.3127896122781,41.3729764244373,-27.6536474577346));
#11421=CARTESIAN_POINT('Ctrl Pts',(48.497021956718,41.5118654613665,-27.7679863269871));
#11422=CARTESIAN_POINT('Ctrl Pts',(48.4985109794233,41.5129859784971,-27.7689128878216));
#11423=CARTESIAN_POINT('Ctrl Pts',(48.5,41.5141044679105,-27.7698418867199));
#11424=CARTESIAN_POINT('Origin',(48.5,54.6122755947453,-11.9999999999999));
#11425=CARTESIAN_POINT('Ctrl Pts',(47.5378994299191,38.9101601847763,-26.2843289888635));
#11426=CARTESIAN_POINT('Ctrl Pts',(47.5689916161584,38.9721723243012,-26.1894802928096));
#11427=CARTESIAN_POINT('Ctrl Pts',(47.6171220217074,39.0145492829462,-26.0896111315549));
#11428=CARTESIAN_POINT('Ctrl Pts',(47.7549681777013,39.0754840945847,-25.8572144843834));
#11429=CARTESIAN_POINT('Ctrl Pts',(47.8576296359838,39.0823902452002,-25.7182913573655));
#11430=CARTESIAN_POINT('Ctrl Pts',(48.1332373666738,39.0334182790756,-25.4052183599782));
#11431=CARTESIAN_POINT('Ctrl Pts',(48.3127896122749,38.9586281370126,-25.2392991703103));
#11432=CARTESIAN_POINT('Ctrl Pts',(48.497021956719,38.8442892677574,-25.1004101333779));
#11433=CARTESIAN_POINT('Ctrl Pts',(48.4985109794223,38.8433627069242,-25.0992896162488));
#11434=CARTESIAN_POINT('Ctrl Pts',(48.5,38.8424337080252,-25.0981711268347));
#11435=CARTESIAN_POINT('Origin',(36.5,54.6122755947453,-11.9999999999999));
#11436=CARTESIAN_POINT('Ctrl Pts',(37.462100570081,38.9101601847763,-26.2843289888635));
#11437=CARTESIAN_POINT('Ctrl Pts',(37.4310083838421,38.9721723243003,-26.1894802928109));
#11438=CARTESIAN_POINT('Ctrl Pts',(37.3828779782939,39.0145492829451,-26.0896111315576));
#11439=CARTESIAN_POINT('Ctrl Pts',(37.2450318223019,39.075484094584,-25.8572144843881));
#11440=CARTESIAN_POINT('Ctrl Pts',(37.1423703640203,39.0823902452002,-25.7182913573708));
#11441=CARTESIAN_POINT('Ctrl Pts',(36.8667626332853,39.0334182790692,-25.4052183599309));
#11442=CARTESIAN_POINT('Ctrl Pts',(36.6872103876556,38.9586281369882,-25.2392991702806));
#11443=CARTESIAN_POINT('Ctrl Pts',(36.502978043283,38.844289267758,-25.1004101333787));
#11444=CARTESIAN_POINT('Ctrl Pts',(36.5014890205765,38.8433627069234,-25.0992896162479));
#11445=CARTESIAN_POINT('Ctrl Pts',(36.5,38.8424337080252,-25.0981711268347));
#11446=CARTESIAN_POINT('Origin',(50.,38.0731731281852,-25.7371063037535));
#11447=CARTESIAN_POINT('Origin',(47.5,38.0731731281855,1.73710630375391));
#11448=CARTESIAN_POINT('Ctrl Pts',(37.462100570081,38.9101601847765,2.2843289888639));
#11449=CARTESIAN_POINT('Ctrl Pts',(37.4310083838418,38.9721723243011,2.1894802928104));
#11450=CARTESIAN_POINT('Ctrl Pts',(37.382877978293,39.0145492829461,2.0896111315562));
#11451=CARTESIAN_POINT('Ctrl Pts',(37.2450318222997,39.0754840945847,1.85721448438531));
#11452=CARTESIAN_POINT('Ctrl Pts',(37.1423703640175,39.0823902452004,1.71829135736766));
#11453=CARTESIAN_POINT('Ctrl Pts',(36.8667626333158,39.0334182790742,1.40521835996645));
#11454=CARTESIAN_POINT('Ctrl Pts',(36.6872103877081,38.9586281370059,1.23929917030242));
#11455=CARTESIAN_POINT('Ctrl Pts',(36.5029780432818,38.844289267758,1.10041013337881));
#11456=CARTESIAN_POINT('Ctrl Pts',(36.5014890205776,38.8433627069243,1.09928961624914));
#11457=CARTESIAN_POINT('Ctrl Pts',(36.5,38.8424337080254,1.09817112683512));
#11458=CARTESIAN_POINT('Ctrl Pts',(47.5378994299191,38.9101601847765,2.2843289888639));
#11459=CARTESIAN_POINT('Ctrl Pts',(47.5689916161585,38.9721723243016,2.18948029280961));
#11460=CARTESIAN_POINT('Ctrl Pts',(47.6171220217078,39.0145492829468,2.08961113155459));
#11461=CARTESIAN_POINT('Ctrl Pts',(47.7549681777024,39.0754840945851,1.85721448438222));
#11462=CARTESIAN_POINT('Ctrl Pts',(47.8576296359852,39.0823902452003,1.71829135736426));
#11463=CARTESIAN_POINT('Ctrl Pts',(48.1332373666565,39.0334182790786,1.40521835999846));
#11464=CARTESIAN_POINT('Ctrl Pts',(48.3127896122453,38.9586281370227,1.23929917032299));
#11465=CARTESIAN_POINT('Ctrl Pts',(48.4970219567186,38.8442892677582,1.10041013337901));
#11466=CARTESIAN_POINT('Ctrl Pts',(48.4985109794219,38.8433627069246,1.09928961624948));
#11467=CARTESIAN_POINT('Ctrl Pts',(48.5,38.8424337080254,1.09817112683513));
#11468=CARTESIAN_POINT('Origin',(48.5,54.6122755947453,-11.9999999999999));
#11469=CARTESIAN_POINT('Ctrl Pts',(47.5378994299191,40.3279466058819,3.70211540996925));
#11470=CARTESIAN_POINT('Ctrl Pts',(47.5689916161576,40.4227953019335,3.64010327044594));
#11471=CARTESIAN_POINT('Ctrl Pts',(47.6171220217051,40.5226644631856,3.59772631180138));
#11472=CARTESIAN_POINT('Ctrl Pts',(47.7549681776959,40.7550611103542,3.53679150016188));
#11473=CARTESIAN_POINT('Ctrl Pts',(47.857629635977,40.8939842373711,3.5298853495454));
#11474=CARTESIAN_POINT('Ctrl Pts',(48.1332373667501,41.2070572348553,3.57885731568198));
#11475=CARTESIAN_POINT('Ctrl Pts',(48.3127896124051,41.3729764244901,3.65364745777795));
#11476=CARTESIAN_POINT('Ctrl Pts',(48.4970219567172,41.5118654613675,3.76798632698816));
#11477=CARTESIAN_POINT('Ctrl Pts',(48.4985109794234,41.5129859784975,3.76891288782207));
#11478=CARTESIAN_POINT('Ctrl Pts',(48.5,41.5141044679107,3.76984188672031));
#11479=CARTESIAN_POINT('Origin',(36.5,54.6122755947453,-11.9999999999999));
#11480=CARTESIAN_POINT('Ctrl Pts',(37.462100570081,40.3279466058819,3.70211540996925));
#11481=CARTESIAN_POINT('Ctrl Pts',(37.4310083838421,40.4227953019343,3.64010327044543));
#11482=CARTESIAN_POINT('Ctrl Pts',(37.3828779782942,40.5226644631872,3.5977263118007));
#11483=CARTESIAN_POINT('Ctrl Pts',(37.2450318223022,40.755061110357,3.53679150016149));
#11484=CARTESIAN_POINT('Ctrl Pts',(37.1423703640206,40.8939842373742,3.52988534954544));
#11485=CARTESIAN_POINT('Ctrl Pts',(36.8667626332747,41.2070572348267,3.57885731567809));
#11486=CARTESIAN_POINT('Ctrl Pts',(36.6872103876371,41.3729764244722,3.65364745776331));
#11487=CARTESIAN_POINT('Ctrl Pts',(36.5029780432816,41.511865461368,3.76798632698854));
#11488=CARTESIAN_POINT('Ctrl Pts',(36.5014890205776,41.5129859784967,3.76891288782145));
#11489=CARTESIAN_POINT('Ctrl Pts',(36.5,41.5141044679107,3.76984188672031));
#11490=CARTESIAN_POINT('Origin',(50.,40.8751692909919,4.53910246656033));
#11491=CARTESIAN_POINT('Origin',(36.,54.6122755947453,-11.9999999999999));
#11492=CARTESIAN_POINT('Origin',(36.,54.6122755947453,7.50000000000008));
#11493=CARTESIAN_POINT('Origin',(49.,54.6122755947453,-11.9999999999999));
#11494=CARTESIAN_POINT('Origin',(49.,54.6122755947453,7.50000000000009));
#11495=CARTESIAN_POINT('Origin',(35.,54.6122755947453,-11.9999999999999));
#11496=CARTESIAN_POINT('',(35.,54.6122755947453,5.50000000000008));
#14103=UNCERTAINTY_MEASURE_WITH_UNIT(LENGTH_MEASURE(0.01),#14126,
'DISTANCE_ACCURACY_VALUE',
'Maximum model space distance between geometric entities at asserted c
onnectivities');
#14112=UNCERTAINTY_MEASURE_WITH_UNIT(LENGTH_MEASURE(0.01),#14126,
'DISTANCE_ACCURACY_VALUE',
'Maximum model space distance between geometric entities at asserted c
onnectivities');
#14116=(
GEOMETRIC_REPRESENTATION_CONTEXT(3)
GLOBAL_UNCERTAINTY_ASSIGNED_CONTEXT((#14103))
GLOBAL_UNIT_ASSIGNED_CONTEXT((#14126,#14128,#14129))
REPRESENTATION_CONTEXT('','3D')
);
#14125=(
GEOMETRIC_REPRESENTATION_CONTEXT(3)
GLOBAL_UNCERTAINTY_ASSIGNED_CONTEXT((#14112))
GLOBAL_UNIT_ASSIGNED_CONTEXT((#14126,#14128,#14129))
REPRESENTATION_CONTEXT('','3D')
);
#14126=(
LENGTH_UNIT()
NAMED_UNIT(*)
SI_UNIT(.MILLI.,.METRE.)
);
#14128=(
NAMED_UNIT(*)
PLANE_ANGLE_UNIT()
SI_UNIT($,.RADIAN.)
);
#14129=(
NAMED_UNIT(*)
SI_UNIT($,.STERADIAN.)
SOLID_ANGLE_UNIT()
);
#14133=SHAPE_DEFINITION_REPRESENTATION(#14145,#14202);
#14145=PRODUCT_DEFINITION_SHAPE('',$,#14215);
#14202=SHAPE_REPRESENTATION('',(#6408),#14116);
#14211=PRODUCT_DEFINITION_CONTEXT('part definition',#14249,'design');
#14215=PRODUCT_DEFINITION('Front Tightener','Front Tightener',#14227,#14211);
#14227=PRODUCT_DEFINITION_FORMATION('',$,#14254);
#14249=APPLICATION_CONTEXT(
'Core Data for Automotive Mechanical Design Process');
#14250=PRODUCT_CONTEXT('part definition',#14249,'mechanical');
#14254=PRODUCT('Front Tightener','Front Tightener',$,(#14250));
#14263=PRESENTATION_STYLE_ASSIGNMENT((#14265));
#14265=SURFACE_STYLE_USAGE(.BOTH.,#14267);
#14267=SURFACE_SIDE_STYLE('',(#14269));
#14269=SURFACE_STYLE_FILL_AREA(#14271);
#14271=FILL_AREA_STYLE('Steel - Satin',(#14273));
#14273=FILL_AREA_STYLE_COLOUR('Steel - Satin',#14275);
#14275=COLOUR_RGB('Steel - Satin',0.627450980392157,0.627450980392157,0.627450980392157);
ENDSEC;
END-ISO-10303-21;
